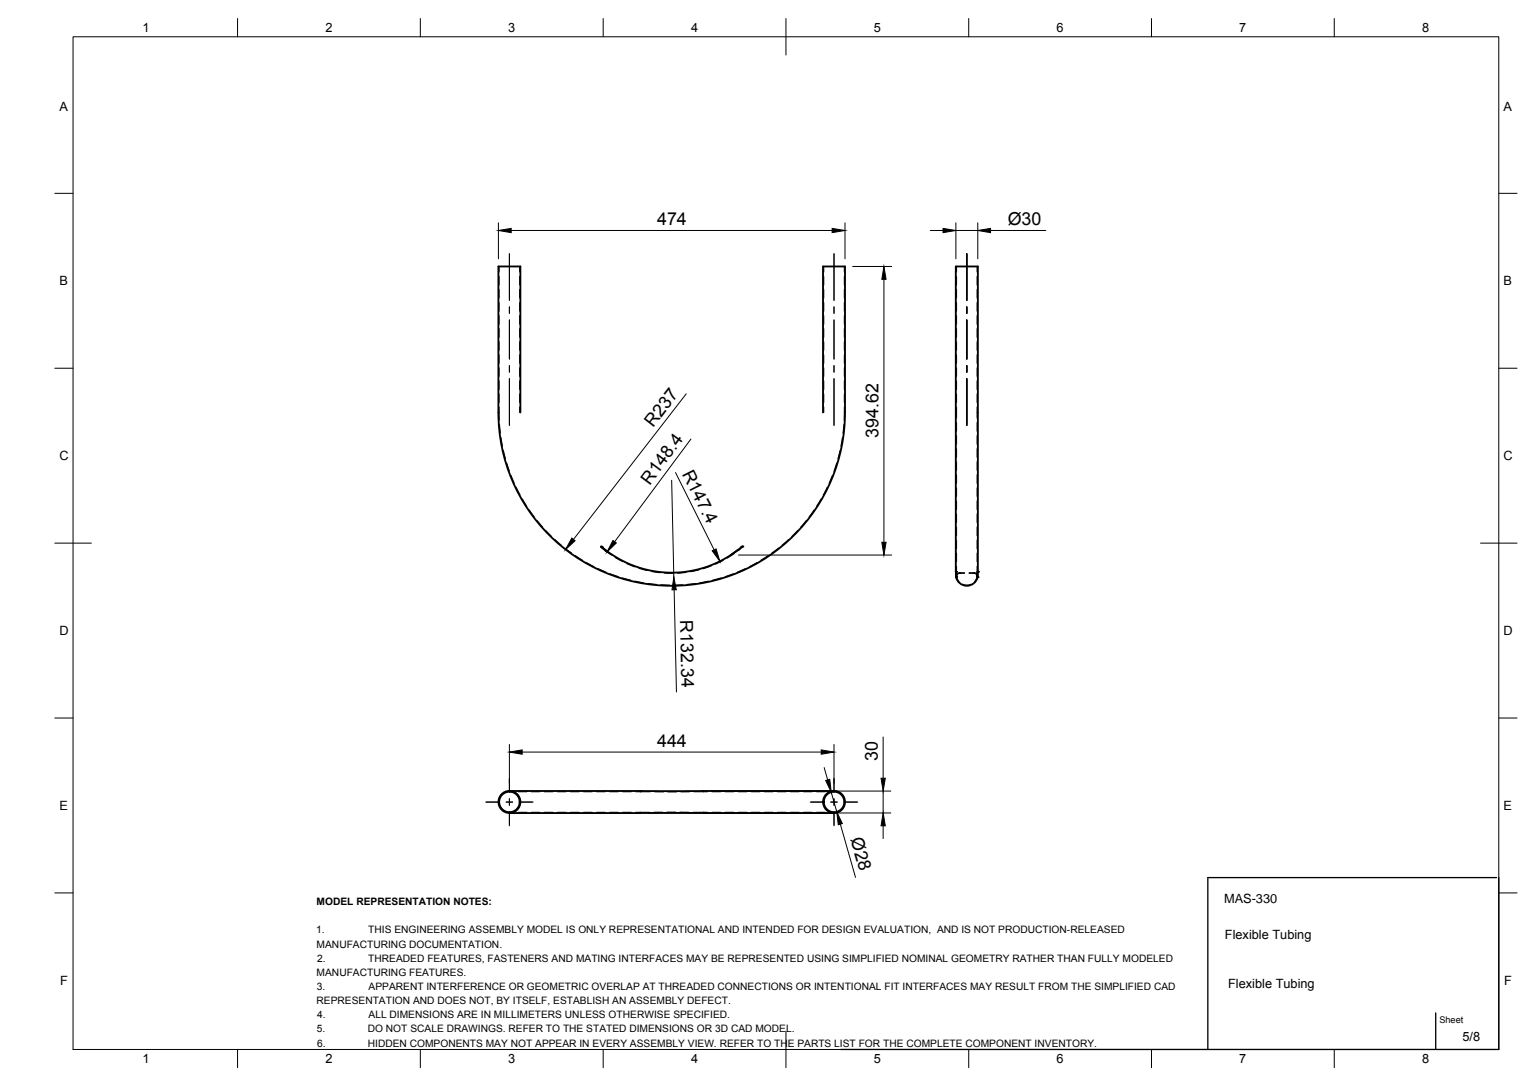
ISO-10303-21;
HEADER;
/* Generated by software containing ST-Developer
 * from STEP Tools, Inc. (www.steptools.com) 
 */

FILE_DESCRIPTION(
/* description */ ('STEP AP214'),
/* implementation_level */ '2;1');

FILE_NAME(
/* name */ 'Flexible Tubing.step',
/* time_stamp */ '2026-10-12T14:05:15-07:00',
/* author */ (''),
/* organization */ (''),
/* preprocessor_version */ 'ST-DEVELOPER v20.2',
/* originating_system */ 'Autodesk Translation Framework v15.15.0.0',
/* authorisation */ '');

FILE_SCHEMA (('AUTOMOTIVE_DESIGN { 1 0 10303 214 3 1 1 }'));
ENDSEC;

DATA;
#10=MECHANICAL_DESIGN_GEOMETRIC_PRESENTATION_REPRESENTATION('',(#284),#39959);
#184=(
BOUNDED_SURFACE()
B_SPLINE_SURFACE(3,2,((#27814,#27815,#27816),(#27817,#27818,#27819),(#27820,
#27821,#27822),(#27823,#27824,#27825),(#27826,#27827,#27828),(#27829,#27830,
#27831),(#27832,#27833,#27834),(#27835,#27836,#27837),(#27838,#27839,#27840),
(#27841,#27842,#27843),(#27844,#27845,#27846),(#27847,#27848,#27849),(#27850,
#27851,#27852),(#27853,#27854,#27855),(#27856,#27857,#27858),(#27859,#27860,
#27861),(#27862,#27863,#27864),(#27865,#27866,#27867),(#27868,#27869,#27870),
(#27871,#27872,#27873),(#27874,#27875,#27876),(#27877,#27878,#27879),(#27880,
#27881,#27882),(#27883,#27884,#27885),(#27886,#27887,#27888),(#27889,#27890,
#27891),(#27892,#27893,#27894),(#27895,#27896,#27897),(#27898,#27899,#27900),
(#27901,#27902,#27903),(#27904,#27905,#27906),(#27907,#27908,#27909),(#27910,
#27911,#27912),(#27913,#27914,#27915),(#27916,#27917,#27918),(#27919,#27920,
#27921),(#27922,#27923,#27924),(#27925,#27926,#27927),(#27928,#27929,#27930),
(#27931,#27932,#27933),(#27934,#27935,#27936),(#27937,#27938,#27939),(#27940,
#27941,#27942),(#27943,#27944,#27945),(#27946,#27947,#27948),(#27949,#27950,
#27951),(#27952,#27953,#27954),(#27955,#27956,#27957),(#27958,#27959,#27960),
(#27961,#27962,#27963),(#27964,#27965,#27966),(#27967,#27968,#27969),(#27970,
#27971,#27972),(#27973,#27974,#27975),(#27976,#27977,#27978),(#27979,#27980,
#27981),(#27982,#27983,#27984),(#27985,#27986,#27987),(#27988,#27989,#27990),
(#27991,#27992,#27993),(#27994,#27995,#27996),(#27997,#27998,#27999),(#28000,
#28001,#28002),(#28003,#28004,#28005),(#28006,#28007,#28008),(#28009,#28010,
#28011),(#28012,#28013,#28014),(#28015,#28016,#28017),(#28018,#28019,#28020),
(#28021,#28022,#28023),(#28024,#28025,#28026),(#28027,#28028,#28029),(#28030,
#28031,#28032),(#28033,#28034,#28035),(#28036,#28037,#28038),(#28039,#28040,
#28041),(#28042,#28043,#28044),(#28045,#28046,#28047),(#28048,#28049,#28050),
(#28051,#28052,#28053),(#28054,#28055,#28056),(#28057,#28058,#28059),(#28060,
#28061,#28062),(#28063,#28064,#28065),(#28066,#28067,#28068),(#28069,#28070,
#28071),(#28072,#28073,#28074),(#28075,#28076,#28077),(#28078,#28079,#28080),
(#28081,#28082,#28083),(#28084,#28085,#28086),(#28087,#28088,#28089),(#28090,
#28091,#28092),(#28093,#28094,#28095),(#28096,#28097,#28098),(#28099,#28100,
#28101)),.UNSPECIFIED.,.F.,.F.,.F.)
B_SPLINE_SURFACE_WITH_KNOTS((4,2,2,2,2,2,2,2,2,2,2,2,2,2,2,2,2,2,2,2,2,
2,2,2,2,2,2,2,2,2,2,2,2,2,2,2,2,2,2,2,2,2,2,2,2,2,2,4),(3,3),(0.22178007142157,
0.223701231496081,0.225435349569694,0.227169467643307,0.228036526680114,
0.228903585716921,0.229770644753727,0.230204174272131,0.230637703790534,
0.231071233308937,0.231504762827341,0.231938292345744,0.232371821864147,
0.232805351382551,0.233238880900954,0.234105939937761,0.234972998974567,
0.235840058011374,0.237574176084987,0.239308294158601,0.241042412232214,
0.242776530305827,0.246244766453054,0.249713002600281,0.256649474894734,
0.260117711041961,0.263585947189187,0.270522419483641,0.277458891778094,
0.291331836367001,0.298268308661454,0.305204780955908,0.319077725544815,
0.332950670133721,0.346823614722628,0.353760087017082,0.360696559311535,
0.374569503900442,0.388442448489349,0.402315393078255,0.409251865372709,
0.416188337667162,0.423124809961615,0.430061282256069,0.433529518403295,
0.436997754550522,0.440465990697749,0.444121268845909),(-0.000187042000933031,
1.00006570533259),.UNSPECIFIED.)
GEOMETRIC_REPRESENTATION_ITEM()
RATIONAL_B_SPLINE_SURFACE(((1.00001671480553,0.955315105954543,1.00000587097346),
(1.00001553678529,0.958464392346589,1.00000545720104),(1.00001436299837,
0.961602361500747,1.00000504491554),(1.00001214511377,0.96753159221984,
1.00000426589711),(1.0000110971902,0.970333081805704,1.00000389782035),
(1.00000903364032,0.975849718381431,1.00000317301105),(1.00000802454064,
0.978547417281528,1.00000281857094),(1.00000657099102,0.982433296228171,
1.0000023080205),(1.0000060954059,0.98370471220148,1.00000214097413),(1.0000051861456,
0.986135503257278,1.000001821602),(1.00000475111726,0.987298495868281,1.00000166880095),
(1.00000393900491,0.989469574341258,1.00000138355144),(1.00000355798186,
0.990488190713896,1.00000124971942),(1.00000307531353,0.991778542734027,
1.00000108018511),(1.00000292909575,0.992169437270804,1.00000102882701),
(1.00000267340501,0.992852993744571,1.0000009390172),(1.00000256420741,
0.993144919550281,1.00000090066221),(1.00000239821197,0.993588687122249,
1.00000084235732),(1.00000234012324,0.993743979916236,1.00000082195401),
(1.00000227962719,0.993905708377709,1.00000080070514),(1.00000227804363,
0.993909941827738,1.00000080014892),(1.00000233322191,0.993762429746366,
1.00000081952996),(1.00000238907502,0.993613113593466,1.00000083914802),
(1.00000255214859,0.993177157271913,1.00000089642662),(1.00000265990449,
0.992889085671756,1.00000093427522),(1.00000291128676,0.992217047317989,
1.00000102257171),(1.00000305564197,0.991831132138118,1.0000010732756),
(1.00000337449658,0.990978715127399,1.00000118527134),(1.00000355003229,
0.990509442879127,1.00000124692718),(1.00000410591494,0.98902336174389,
1.00000144217757),(1.00000451382822,0.987932857764997,1.00000158545462),
(1.0000053771532,0.985624868901155,1.00000188869225),(1.00000583381796,
0.984404034076013,1.00000204909296),(1.00000677789068,0.981880176447102,
1.00000238069275),(1.00000726052111,0.980589925744053,1.00000255021374),
(1.00000873064634,0.976659734042192,1.00000306658626),(1.00000973994235,
0.973961510289341,1.00000342109532),(1.00001179196766,0.968475683150999,
1.00000414185669),(1.00001283513645,0.96568690486921,1.00000450826337),
(1.00001494361968,0.960050144712234,1.00000524885524),(1.00001601138312,
0.95719561576597,1.00000562390063),(1.00001814845983,0.951482414616923,
1.00000637453578),(1.00001921796653,0.948623225275015,1.00000675019349),
(1.00002242616289,0.940046522775516,1.00000787705289),(1.00002456438731,
0.934330253373406,1.00000862809117),(1.00002882929853,0.922928558871327,
1.00001012611521),(1.00003095610456,0.91724281507434,1.00001087314285),
(1.00003730979308,0.900257041725582,1.00001310483718),(1.00004150973089,
0.889029045332982,1.00001458003971),(1.00004772883642,0.872403062390114,
1.00001676446258),(1.00004978850184,0.866896810424999,1.00001748790749),
(1.00005387724354,0.855966082598523,1.00001892405307),(1.00005590801946,
0.850537063013456,1.00001963735072),(1.00006192256307,0.834457950174723,
1.00002174992247),(1.00006583638793,0.823994840153908,1.00002312462957),
(1.00007345352895,0.803631388209101,1.00002580010388),(1.00007715685939,
0.793731008091671,1.0000271008761),(1.00008791765573,0.764963395833388,
1.00003088054016),(1.00009462794849,0.747024286693254,1.00003323748955),
(1.00010382896234,0.722426553366422,1.00003646928952),(1.00010675138937,
0.71461381858396,1.00003749577419),(1.00011227304363,0.699852382375851,
1.00003943522156),(1.00011487430917,0.692898231787275,1.00004034890021),
(1.00012212392104,0.673517321968125,1.00004289528215),(1.00012616942783,
0.662702177158641,1.00004431624172),(1.0001325032316,0.645769563161906,
1.00004654095165),(1.00013478994257,0.639656333948816,1.00004734414493),
(1.0001374601242,0.632517944987879,1.00004828202993),(1.00013784258632,
0.631495481447842,1.00004841636742),(1.00013694003487,0.63390833726827,
1.00004809935173),(1.00013639387768,0.635368418638627,1.00004790751735),
(1.00013481186227,0.63959773443293,1.00004735184409),(1.00013378125052,
0.642352943082953,1.000046989848),(1.00013001435257,0.652423262814007,1.00004566674808),
(1.00012660145365,0.661547211425516,1.00004446798815),(1.00011821711893,
0.683961657570758,1.00004152304174),(1.00011324709426,0.697248382663264,
1.0000397773509),(1.00010199064016,0.727341072498234,1.00003582359008),
(1.00009570502111,0.744144870834123,1.00003361580473),(1.00008544083,0.771584872526209,
1.00003001057023),(1.00008187300066,0.781123007795138,1.00002875739195),
(1.000074536318,0.800736690215974,1.00002618042693),(1.00007076318398,0.810823681264022,
1.00002485513662),(1.000063033788,0.831487232491117,1.00002214023345),(1.0000590774879,
0.84206389463353,1.00002075060717),(1.00005100479812,0.863645197935074,
1.00001791512414),(1.00004688833189,0.874650043707415,1.0000164692405),
(1.00004060950573,0.891435682115803,1.00001426384112),(1.00003849870446,
0.897078639254129,1.00001352243505),(1.00003426394995,0.908399713630422,
1.00001203500336),(1.00003213787031,0.914083515546979,1.00001128823086),
(1.00002787459407,0.925480839114136,1.00000979078109),(1.00002573731916,
0.931194570120134,1.00000904007632),(1.00002134529738,0.94293607843551,
1.00000749740547),(1.00001909036436,0.94896435336469,1.000006705374),(1.00001684310806,
0.954972105552579,1.00000591603894)))
REPRESENTATION_ITEM('')
SURFACE()
);
#185=(
BOUNDED_SURFACE()
B_SPLINE_SURFACE(3,2,((#28385,#28386,#28387),(#28388,#28389,#28390),(#28391,
#28392,#28393),(#28394,#28395,#28396),(#28397,#28398,#28399),(#28400,#28401,
#28402),(#28403,#28404,#28405),(#28406,#28407,#28408),(#28409,#28410,#28411),
(#28412,#28413,#28414),(#28415,#28416,#28417),(#28418,#28419,#28420),(#28421,
#28422,#28423),(#28424,#28425,#28426),(#28427,#28428,#28429),(#28430,#28431,
#28432),(#28433,#28434,#28435),(#28436,#28437,#28438),(#28439,#28440,#28441),
(#28442,#28443,#28444),(#28445,#28446,#28447),(#28448,#28449,#28450),(#28451,
#28452,#28453),(#28454,#28455,#28456),(#28457,#28458,#28459),(#28460,#28461,
#28462),(#28463,#28464,#28465),(#28466,#28467,#28468),(#28469,#28470,#28471),
(#28472,#28473,#28474),(#28475,#28476,#28477),(#28478,#28479,#28480),(#28481,
#28482,#28483),(#28484,#28485,#28486),(#28487,#28488,#28489),(#28490,#28491,
#28492),(#28493,#28494,#28495),(#28496,#28497,#28498),(#28499,#28500,#28501),
(#28502,#28503,#28504),(#28505,#28506,#28507),(#28508,#28509,#28510),(#28511,
#28512,#28513),(#28514,#28515,#28516),(#28517,#28518,#28519),(#28520,#28521,
#28522),(#28523,#28524,#28525),(#28526,#28527,#28528),(#28529,#28530,#28531),
(#28532,#28533,#28534),(#28535,#28536,#28537),(#28538,#28539,#28540),(#28541,
#28542,#28543),(#28544,#28545,#28546),(#28547,#28548,#28549),(#28550,#28551,
#28552),(#28553,#28554,#28555),(#28556,#28557,#28558),(#28559,#28560,#28561),
(#28562,#28563,#28564),(#28565,#28566,#28567),(#28568,#28569,#28570),(#28571,
#28572,#28573),(#28574,#28575,#28576),(#28577,#28578,#28579),(#28580,#28581,
#28582),(#28583,#28584,#28585),(#28586,#28587,#28588),(#28589,#28590,#28591),
(#28592,#28593,#28594),(#28595,#28596,#28597),(#28598,#28599,#28600),(#28601,
#28602,#28603),(#28604,#28605,#28606),(#28607,#28608,#28609),(#28610,#28611,
#28612),(#28613,#28614,#28615),(#28616,#28617,#28618),(#28619,#28620,#28621),
(#28622,#28623,#28624),(#28625,#28626,#28627),(#28628,#28629,#28630),(#28631,
#28632,#28633),(#28634,#28635,#28636),(#28637,#28638,#28639),(#28640,#28641,
#28642),(#28643,#28644,#28645),(#28646,#28647,#28648),(#28649,#28650,#28651),
(#28652,#28653,#28654),(#28655,#28656,#28657),(#28658,#28659,#28660),(#28661,
#28662,#28663),(#28664,#28665,#28666),(#28667,#28668,#28669),(#28670,#28671,
#28672),(#28673,#28674,#28675),(#28676,#28677,#28678),(#28679,#28680,#28681),
(#28682,#28683,#28684),(#28685,#28686,#28687),(#28688,#28689,#28690)),
 .UNSPECIFIED.,.F.,.F.,.F.)
B_SPLINE_SURFACE_WITH_KNOTS((4,2,2,2,2,2,2,2,2,2,2,2,2,2,2,2,2,2,2,2,2,
2,2,2,2,2,2,2,2,2,2,2,2,2,2,2,2,2,2,2,2,2,2,2,2,2,2,2,2,2,4),(3,3),(0.,
0.00173411807361341,0.00346823614722682,0.00520235422084023,0.00606941325764693,
0.00693647229445363,0.00780353133126034,0.00867059036806704,0.00910411988647039,
0.00953764940487375,0.0099711789232771,0.0104047084416805,0.0108382379600838,
0.0112717674784872,0.0117052969968905,0.0121388265152939,0.0130058855521006,
0.0138729445889073,0.0156070626625207,0.0173411807361341,0.0190752988097475,
0.0208094168833609,0.0242776530305877,0.0277458891778145,0.0346823614722682,
0.038150597619495,0.0416188337667218,0.0485553060611754,0.0554917783556291,
0.0693647229445363,0.0832376675334436,0.0867059036806704,0.0901741398278972,
0.0971106121223509,0.110983556711258,0.124856501300165,0.131792973594619,
0.135261209741846,0.138729445889073,0.15260239047798,0.166475335066887,
0.180348279655794,0.183816515803021,0.187284751950248,0.194221224244702,
0.201157696539155,0.208094168833609,0.211562404980836,0.215030641128063,
0.218498877275289,0.222038288720656),(0.,1.00007117529817),
 .UNSPECIFIED.)
GEOMETRIC_REPRESENTATION_ITEM()
RATIONAL_B_SPLINE_SURFACE(((1.,0.954058032824739,1.00000653986642),(1.,
0.956926189621845,1.00000613158259),(1.,0.959774945923169,1.00000572606044),
(1.,0.965414443781637,1.00000492327455),(1.,0.968205662454782,1.00000452594291),
(1.,0.973699562224279,1.000003743883),(1.,0.976403365991766,1.00000335899492),
(1.,0.98034605056057,1.00000279775142),(1.,0.981641163134558,1.00000261339138),
(1.,0.984176833060148,1.00000225243725),(1.,0.985416251002957,1.00000207600537),
(1.,0.987758111159059,1.00000174264018),(1.,0.988874643995945,1.00000158370106),
(1.,0.99087726268354,1.0000012986271),(1.,0.991757284799027,1.00000117335542),
(1.,0.992797059568252,1.00000102534287),(1.,0.993098523876015,1.00000098242924),
(1.,0.993562924435804,1.00000091632155),(1.,0.993726976585977,1.00000089296862),
(1.,0.9939034030842,1.00000086785421),(1.,0.993913510674876,1.00000086641539),
(1.,0.993776600284822,1.00000088590466),(1.,0.993631545571422,1.00000090655329),
(1.,0.993199734841636,1.0000009680218),(1.,0.992914845213595,1.00000100857601),
(1.,0.99224575536465,1.00000110382135),(1.,0.991859782611137,1.0000011587648),
(1.,0.991003776450707,1.00000128061779),(1.,0.990532224611597,1.00000134774347),
(1.,0.989541347388611,1.00000148879544),(1.,0.98901957113283,1.0000015630706),
(1.,0.987391710342441,1.00000179479755),(1.,0.986223928377901,1.00000196103201),
(1.,0.983775371631144,1.00000230958552),(1.,0.982504716794789,1.000002490464),
(1.,0.97863152044244,1.00000304181581),(1.,0.975951927850889,1.00000342325741),
(1.,0.970485088654407,1.00000420146523),(1.,0.967696119306073,1.00000459847668),
(1.,0.962047336054619,1.00000540258435),(1.,0.959183960598246,1.00000581018755),
(1.,0.953462458079452,1.00000662464684),(1.,0.950596652764379,1.00000703259594),
(1.,0.941994603975872,1.00000825710271),(1.,0.936254194204132,1.00000907425347),
(1.,0.924794890941365,1.00001070549212),(1.,0.919075593477731,1.00001151963753),
(1.,0.901978842716718,1.00001395337019),(1.,0.890663248710558,1.00001556415175),
(1.,0.8738935874927,1.00001795132302),(1.,0.868330212597956,1.00001874327276),
(1.,0.857329904873204,1.00002030917312),(1.,0.851890471291245,1.00002108347973),
(1.,0.835762777169572,1.00002337926661),(1.,0.825264842647475,1.00002487365385),
(1.,0.804827719776929,1.00002778289048),(1.,0.794888487743137,1.00002919774608),
(1.,0.765999443480927,1.00003331011876),(1.,0.747972792915185,1.00003587622322),
(1.,0.714994849965956,1.00004057065307),(1.,0.700044230979255,1.00004269888259),
(1.,0.683764200151961,1.00004501635469),(1.,0.680628844586273,1.00004546267443),
(1.,0.674640520726457,1.0000463151159),(1.,0.671783516007252,1.00004672181222),
(1.,0.663635510374337,1.00004788168568),(1.,0.658767677401333,1.00004857462461),
(1.,0.645945349063695,1.0000503998907),(1.,0.639777818633445,1.00005127784233),
(1.,0.632581312956382,1.00005230226921),(1.,0.631555065114158,1.0000524483562),
(1.,0.63399275055746,1.00005210135022),(1.,0.635466148812585,1.0000518916111),
(1.,0.638664401233599,1.00005143633796),(1.,0.639895676582775,1.00005126106518),
(1.,0.642669442581869,1.00005086621794),(1.,0.644213120868507,1.00005064647441),
(1.,0.652691129180967,1.00004943962487),(1.,0.661906311274784,1.00004812783821),
(1.,0.684528677277457,1.00004490753092),(1.,0.697932027791846,1.00004299955598),
(1.,0.728267963131221,1.00003868121749),(1.,0.745198393491031,1.00003627116063),
(1.,0.768222924620666,1.0000329936049),(1.,0.772921247385803,1.00003232479585),
(1.,0.782497618983893,1.00003096159364),(1.,0.787373779802698,1.00003026746924),
(1.,0.802194699878368,1.00002815770243),(1.,0.812351834256105,1.00002671182829),
(1.,0.833145675250053,1.00002375181263),(1.,0.843782502229831,1.00002223765397),
(1.,0.86547121370724,1.00001915025295),(1.,0.876523345831396,1.00001757697535),
(1.,0.893367253742941,1.00001517923502),(1.,0.899026187982997,1.00001437368235),
(1.,0.910424400977938,1.00001275113994),(1.,0.916164825311843,1.00001193398711),
(1.,0.927638312474702,1.00001030072937),(1.,0.933380131170828,1.00000948337806),
(1.,0.944959178856698,1.00000783509371),(1.,0.950796193416408,1.00000700419121),
(1.,0.95659226878001,1.00000617911642)))
REPRESENTATION_ITEM('')
SURFACE()
);
#186=(
BOUNDED_SURFACE()
B_SPLINE_SURFACE(3,2,((#29356,#29357,#29358),(#29359,#29360,#29361),(#29362,
#29363,#29364),(#29365,#29366,#29367),(#29368,#29369,#29370),(#29371,#29372,
#29373),(#29374,#29375,#29376),(#29377,#29378,#29379),(#29380,#29381,#29382),
(#29383,#29384,#29385),(#29386,#29387,#29388),(#29389,#29390,#29391),(#29392,
#29393,#29394),(#29395,#29396,#29397),(#29398,#29399,#29400),(#29401,#29402,
#29403),(#29404,#29405,#29406),(#29407,#29408,#29409),(#29410,#29411,#29412),
(#29413,#29414,#29415),(#29416,#29417,#29418),(#29419,#29420,#29421),(#29422,
#29423,#29424),(#29425,#29426,#29427),(#29428,#29429,#29430),(#29431,#29432,
#29433),(#29434,#29435,#29436),(#29437,#29438,#29439),(#29440,#29441,#29442),
(#29443,#29444,#29445),(#29446,#29447,#29448),(#29449,#29450,#29451),(#29452,
#29453,#29454),(#29455,#29456,#29457),(#29458,#29459,#29460),(#29461,#29462,
#29463),(#29464,#29465,#29466),(#29467,#29468,#29469),(#29470,#29471,#29472),
(#29473,#29474,#29475),(#29476,#29477,#29478),(#29479,#29480,#29481),(#29482,
#29483,#29484),(#29485,#29486,#29487),(#29488,#29489,#29490),(#29491,#29492,
#29493),(#29494,#29495,#29496),(#29497,#29498,#29499),(#29500,#29501,#29502),
(#29503,#29504,#29505),(#29506,#29507,#29508),(#29509,#29510,#29511),(#29512,
#29513,#29514),(#29515,#29516,#29517),(#29518,#29519,#29520),(#29521,#29522,
#29523),(#29524,#29525,#29526),(#29527,#29528,#29529),(#29530,#29531,#29532),
(#29533,#29534,#29535),(#29536,#29537,#29538),(#29539,#29540,#29541),(#29542,
#29543,#29544),(#29545,#29546,#29547),(#29548,#29549,#29550),(#29551,#29552,
#29553),(#29554,#29555,#29556),(#29557,#29558,#29559),(#29560,#29561,#29562),
(#29563,#29564,#29565),(#29566,#29567,#29568),(#29569,#29570,#29571),(#29572,
#29573,#29574),(#29575,#29576,#29577),(#29578,#29579,#29580),(#29581,#29582,
#29583),(#29584,#29585,#29586),(#29587,#29588,#29589),(#29590,#29591,#29592),
(#29593,#29594,#29595),(#29596,#29597,#29598),(#29599,#29600,#29601),(#29602,
#29603,#29604),(#29605,#29606,#29607),(#29608,#29609,#29610),(#29611,#29612,
#29613),(#29614,#29615,#29616),(#29617,#29618,#29619),(#29620,#29621,#29622),
(#29623,#29624,#29625),(#29626,#29627,#29628),(#29629,#29630,#29631),(#29632,
#29633,#29634),(#29635,#29636,#29637),(#29638,#29639,#29640),(#29641,#29642,
#29643)),.UNSPECIFIED.,.F.,.F.,.F.)
B_SPLINE_SURFACE_WITH_KNOTS((4,2,2,2,2,2,2,2,2,2,2,2,2,2,2,2,2,2,2,2,2,
2,2,2,2,2,2,2,2,2,2,2,2,2,2,2,2,2,2,2,2,2,2,2,2,2,2,4),(3,3),(0.221817496371262,
0.223701231496101,0.225435349569714,0.227169467643327,0.228036526680134,
0.228903585716941,0.229770644753747,0.23020417427215,0.230637703790554,
0.231071233308957,0.23150476282736,0.231938292345764,0.232371821864167,
0.23280535138257,0.233238880900974,0.23410593993778,0.234972998974587,0.235840058011393,
0.237574176085006,0.23930829415862,0.241042412232233,0.242776530305846,
0.246244766453072,0.249713002600299,0.256649474894752,0.260117711041978,
0.263585947189204,0.270522419483657,0.27745889177811,0.291331836367015,
0.298268308661468,0.305204780955921,0.319077725544826,0.332950670133732,
0.346823614722637,0.35376008701709,0.360696559311543,0.374569503900448,
0.388442448489354,0.402315393078259,0.409251865372712,0.416188337667165,
0.423124809961617,0.43006128225607,0.433529518403296,0.436997754550523,
0.440465990697749,0.44408384389623),(-0.000149617051253964,1.00007479383841),
 .UNSPECIFIED.)
GEOMETRIC_REPRESENTATION_ITEM()
RATIONAL_B_SPLINE_SURFACE(((1.00001331480133,0.955500401761319,1.00000665559565),
(1.00001239101105,0.958587815164465,1.00000619382575),(1.00001147053421,
0.961664154694889,1.00000573371211),(1.0000097146529,0.967532512098177,
1.00000485600949),(1.00000887643813,0.970333922314243,1.00000443701574),
(1.00000722584258,0.975850402594055,1.00000361194172),(1.00000641868232,
0.978548025065446,1.00000320847102),(1.00000525601474,0.982433793918799,
1.00000262729484),(1.00000487560295,0.983705173871199,1.00000243714052),
(1.00000414830239,0.986135896059087,1.00000207358883),(1.00000380033123,
0.98729885572081,1.00000189965042),(1.00000315073751,0.989469872683854,
1.00000157494163),(1.00000284596418,0.990488460197697,1.00000142259628),
(1.00000245988668,0.991778775660097,1.00000122960987),(1.00000234292976,
0.992169659122265,1.00000117114726),(1.00000213840745,0.992853196229914,
1.00000106891383),(1.0000020510623,0.993145113764892,1.0000010252531),(1.0000019182856,
0.993588868764268,1.00000095888275),(1.0000018718215,0.993744157158601,
1.000000935657),(1.00000182343182,0.993905881037986,1.00000091146872),(1.00000182216515,
0.993910114368128,1.00000091083556),(1.00000186630125,0.993762606465926,
1.00000093289762),(1.00000191097712,0.993613294543411,1.0000009552295),
(1.00000204141667,0.993177350573097,1.00000102043159),(1.00000212760863,
0.992889287134443,1.00000106351589),(1.00000232868468,0.992217267820518,
1.00000116402665),(1.00000244415175,0.991831363574199,1.00000122174454),
(1.00000269919769,0.990978970713684,1.00000134923293),(1.00000283960547,
0.990509711760598,1.00000141941779),(1.00000328424576,0.989023672728241,
1.00000164167766),(1.00000361052809,0.987933199644816,1.00000180477459),
(1.00000430108584,0.985625276169944,1.00000214995985),(1.00000466636358,
0.984404475932691,1.0000023325492),(1.00000542150997,0.981880689808502,
1.00000271002002),(1.00000580755716,0.980590475660211,1.00000290299128),
(1.00000698348326,0.976660395306211,1.00000349079492),(1.00000779080056,
0.973962247998255,1.00000389434413),(1.00000943217783,0.968476576281456,
1.00000471481025),(1.00001026658934,0.965687877010012,1.00000513190289),
(1.00001195312625,0.960051276550606,1.00000597494271),(1.00001280721057,
0.957196828477568,1.00000640186909),(1.00001451661888,0.951483789191777,
1.00000725634151),(1.00001537209761,0.948624680855099,1.0000076839649),
(1.00001793827481,0.940048221346092,1.00000896670562),(1.00001964860115,
0.934332113895509,1.00000982163693),(1.00002306002512,0.922930742418279,
1.00001152688645),(1.0000247612181,0.917245159708875,1.00001237725232),
(1.00002984341657,0.900259867589174,1.00001491766259),(1.0000332028695,
0.889032189306294,1.00001659693363),(1.00003817741751,0.872406677399274,
1.00001908353327),(1.00003982490596,0.866900581435969,1.00001990705415),
(1.00004309541517,0.855970163292049,1.00002154186539),(1.00004471979543,
0.850541297518764,1.00002235383532),(1.00004953071814,0.834462640227989,
1.00002475864448),(1.00005266131459,0.823999826640663,1.00002632351831),
(1.00005875412544,0.803636951622608,1.00002936909777),(1.00006171635128,
0.79373685199774,1.00003084980912),(1.00007032371416,0.764970054768136,
1.00003515232371),(1.00007569115378,0.747031453875889,1.00003783531589),
(1.00008305087536,0.722434417430132,1.00004151417897),(1.00008538847094,
0.714621904001906,1.00004268265986),(1.00008980514053,0.699860885997467,
1.00004489039591),(1.00009188584494,0.692906932438445,1.00004593046605),
(1.00009768467601,0.673526571699192,1.00004882909547),(1.0001009206024,
0.662711733315835,1.00005044661999),(1.00010598689542,0.645779599024357,
1.0000529790797),(1.00010781599343,0.639666543011674,1.00005389338074),
(1.00010995182255,0.632528356305523,1.00005496100576),(1.00011025774696,
0.631505921714365,1.00005511392649),(1.00010953581267,0.633918709193333,
1.00005475305721),(1.00010909895159,0.635378749188762,1.0000545346859),
(1.00010783352659,0.639607945165404,1.00005390214494),(1.00010700915923,
0.642363075750804,1.00005349007302),(1.00010399608691,0.652433110183563,
1.00005198394532),(1.00010126617189,0.661556800302084,1.00005061935789),
(1.00009455969692,0.683970611397211,1.00004726702956),(1.00009058426569,
0.697256960064698,1.00004527985287),(1.0000815804353,0.727348797329703,
1.00004077915827),(1.00007655268435,0.744152119587061,1.00003826596438),
(1.00006834254686,0.77159134386594,1.00003416200863),(1.00006548870585,
0.781129208903971,1.00003273547501),(1.00005962022847,0.800742335641159,
1.00002980203187),(1.00005660216804,0.810829040908275,1.0000282934108),
(1.0000504195665,0.831492006708402,1.00002520294817),(1.00004725499489,
0.842068369196021,1.00002362109137),(1.00004079779896,0.863649061069833,
1.00002039336876),(1.00003750511341,0.874653595057445,1.00001874747236),
(1.00003248279597,0.891438757903646,1.00001623699448),(1.00003079440489,
0.897081555169982,1.00001539302783),(1.00002740710273,0.908402308800912,
1.00001369983595),(1.00002570649076,0.914085949687904,1.0000128497605),
(1.00002229637459,0.925482950352643,1.00001114516471),(1.00002058680775,
0.931196519480498,1.00001029061304),(1.00001709216721,0.942876010290598,
1.00000854376652),(1.00001530696519,0.948842360878052,1.00000765140752),
(1.00001352770684,0.954788847051718,1.00000676201955)))
REPRESENTATION_ITEM('')
SURFACE()
);
#187=(
BOUNDED_SURFACE()
B_SPLINE_SURFACE(3,2,((#30000,#30001,#30002),(#30003,#30004,#30005),(#30006,
#30007,#30008),(#30009,#30010,#30011),(#30012,#30013,#30014),(#30015,#30016,
#30017),(#30018,#30019,#30020),(#30021,#30022,#30023),(#30024,#30025,#30026),
(#30027,#30028,#30029),(#30030,#30031,#30032),(#30033,#30034,#30035),(#30036,
#30037,#30038),(#30039,#30040,#30041),(#30042,#30043,#30044),(#30045,#30046,
#30047),(#30048,#30049,#30050),(#30051,#30052,#30053),(#30054,#30055,#30056),
(#30057,#30058,#30059),(#30060,#30061,#30062),(#30063,#30064,#30065),(#30066,
#30067,#30068),(#30069,#30070,#30071),(#30072,#30073,#30074),(#30075,#30076,
#30077),(#30078,#30079,#30080),(#30081,#30082,#30083),(#30084,#30085,#30086),
(#30087,#30088,#30089),(#30090,#30091,#30092),(#30093,#30094,#30095),(#30096,
#30097,#30098),(#30099,#30100,#30101),(#30102,#30103,#30104),(#30105,#30106,
#30107),(#30108,#30109,#30110),(#30111,#30112,#30113),(#30114,#30115,#30116),
(#30117,#30118,#30119),(#30120,#30121,#30122),(#30123,#30124,#30125),(#30126,
#30127,#30128),(#30129,#30130,#30131),(#30132,#30133,#30134),(#30135,#30136,
#30137),(#30138,#30139,#30140),(#30141,#30142,#30143),(#30144,#30145,#30146),
(#30147,#30148,#30149),(#30150,#30151,#30152),(#30153,#30154,#30155),(#30156,
#30157,#30158),(#30159,#30160,#30161),(#30162,#30163,#30164),(#30165,#30166,
#30167),(#30168,#30169,#30170),(#30171,#30172,#30173),(#30174,#30175,#30176),
(#30177,#30178,#30179),(#30180,#30181,#30182),(#30183,#30184,#30185),(#30186,
#30187,#30188),(#30189,#30190,#30191),(#30192,#30193,#30194),(#30195,#30196,
#30197),(#30198,#30199,#30200),(#30201,#30202,#30203),(#30204,#30205,#30206),
(#30207,#30208,#30209),(#30210,#30211,#30212),(#30213,#30214,#30215),(#30216,
#30217,#30218),(#30219,#30220,#30221),(#30222,#30223,#30224),(#30225,#30226,
#30227),(#30228,#30229,#30230),(#30231,#30232,#30233),(#30234,#30235,#30236),
(#30237,#30238,#30239),(#30240,#30241,#30242),(#30243,#30244,#30245),(#30246,
#30247,#30248),(#30249,#30250,#30251),(#30252,#30253,#30254),(#30255,#30256,
#30257),(#30258,#30259,#30260),(#30261,#30262,#30263),(#30264,#30265,#30266),
(#30267,#30268,#30269),(#30270,#30271,#30272),(#30273,#30274,#30275),(#30276,
#30277,#30278),(#30279,#30280,#30281),(#30282,#30283,#30284),(#30285,#30286,
#30287),(#30288,#30289,#30290),(#30291,#30292,#30293),(#30294,#30295,#30296),
(#30297,#30298,#30299)),.UNSPECIFIED.,.F.,.F.,.F.)
B_SPLINE_SURFACE_WITH_KNOTS((4,2,2,2,2,2,2,2,2,2,2,2,2,2,2,2,2,2,2,2,2,
2,2,2,2,2,2,2,2,2,2,2,2,2,2,2,2,2,2,2,2,2,2,2,2,2,2,2,2,4),(3,3),(-0.000102234541641357,
0.00346823614722661,0.00520235422083992,0.00606941325764658,0.00693647229445323,
0.00780353133125988,0.00867059036806653,0.00910411988646986,0.00953764940487319,
0.00997117892327651,0.0104047084416798,0.0108382379600832,0.0112717674784865,
0.0117052969968898,0.0121388265152932,0.0130058855520998,0.0138729445889065,
0.0156070626625198,0.0173411807361331,0.0190752988097464,0.0208094168833597,
0.0242776530305863,0.0277458891778129,0.0346823614722661,0.0381505976194928,
0.0416188337667194,0.0485553060611726,0.0554917783556258,0.0693647229445323,
0.0832376675334387,0.0867059036806654,0.090174139827892,0.0971106121223452,
0.110983556711252,0.124856501300158,0.131792973594611,0.135261209741838,
0.138729445889065,0.152602390477971,0.166475335066877,0.180348279655784,
0.183816515803011,0.187284751950237,0.19422122424469,0.201157696539144,
0.208094168833597,0.211562404980823,0.21503064112805,0.218498877275277,
0.22202653747512),(0.,1.00010223454164),.UNSPECIFIED.)
GEOMETRIC_REPRESENTATION_ITEM()
RATIONAL_B_SPLINE_SURFACE(((1.,0.953549407570009,1.00000949771005),(1.,
0.959455865791245,1.00000829002195),(1.,0.965295688977991,1.00000709595866),
(1.,0.973698745410201,1.00000537779342),(1.,0.976402633150356,1.00000482493197),
(1.,0.980345440167197,1.00000401874983),(1.,0.981640592963782,1.00000375393113),
(1.,0.9841763416393,1.00000323544892),(1.,0.985415798074981,1.0000029820184),
(1.,0.987757730962312,1.00000250316553),(1.,0.988874298475363,1.00000227486199),
(1.,0.990876979358417,1.00000186537567),(1.,0.991757028804683,1.00000168543276),
(1.,0.992796835866325,1.00000147282437),(1.,0.993098309536668,1.00000141118232),
(1.,0.99356272451931,1.00000131622382),(1.,0.993726781764482,1.00000128267918),
(1.,0.993903213741988,1.0000012466043),(1.,0.993913321646593,1.00000124453754),
(1.,0.993776407004476,1.00000127253235),(1.,0.993631347786124,1.00000130219248),
(1.,0.993199523645578,1.00000139048717),(1.,0.992914625169687,1.0000014487401),
(1.,0.992245514540845,1.00000158555253),(1.,0.99185952980013,1.00000166447448),
(1.,0.991003497054706,1.00000183950671),(1.,0.990531930570611,1.00000193592748),
(1.,0.989541022573869,1.00000213853753),(1.,0.989019230113308,1.00000224522795),
(1.,0.987391318766343,1.00000257808549),(1.,0.986223500534092,1.00000281686822),
(1.,0.983774867742231,1.00000331753792),(1.,0.982504173443108,1.00000357735562),
(1.,0.978630856801064,1.00000436932912),(1.,0.975951180989188,1.00000491723998),
(1.,0.970484172008772,1.00000603507429),(1.,0.96769511604352,1.00000660535001),
(1.,0.96204615735736,1.00000776038741),(1.,0.959182692973428,1.00000834587735),
(1.,0.953461012761225,1.00000951578406),(1.,0.950595118442744,1.00001010177084),
(1.,0.941992802500896,1.0000118606785),(1.,0.936252214448483,1.00001303445127),
(1.,0.924792555293885,1.00001537759728),(1.,0.919073080205329,1.0000165470531),
(1.,0.901975798471311,1.00002004291863),(1.,0.890659853037534,1.00002235667962),
(1.,0.873889671000668,1.00002578566336),(1.,0.868326123324781,1.00002692323686),
(1.,0.857325473963624,1.00002917252955),(1.,0.851885871450147,1.00003028476009),
(1.,0.83575767644592,1.00003358247733),(1.,0.825259415892199,1.00003572904704),
(1.,0.804821658304747,1.0000399079366),(1.,0.794882117587898,1.00004194026538),
(1.,0.765992176118451,1.00004784736523),(1.,0.74796496570046,1.00005153337242),
(1.,0.714985998549083,1.0000582765516),(1.,0.700034915249734,1.0000613335859),
(1.,0.683754378804637,1.00006466245226),(1.,0.680618925863469,1.00006530355545),
(1.,0.674630416028701,1.00006652802056),(1.,0.671773322578567,1.00006711220784),
(1.,0.663625063888358,1.00006877827483),(1.,0.658757079736063,1.00006977362708),
(1.,0.645934353180302,1.00007239547823),(1.,0.63976663119061,1.00007365658669),
(1.,0.632569902032773,1.0000751280953),(1.,0.631543622312258,1.00007533793778),
(1.,0.633981383455941,1.00007483949099),(1.,0.63545482746786,1.00007453821724),
(1.,0.638653179224426,1.00007388425319),(1.,0.639884492811753,1.00007363248763),
(1.,0.642658344954122,1.00007306532063),(1.,0.644202071179115,1.00007274967634),
(1.,0.652680342816058,1.00007101613191),(1.,0.661895811073965,1.00006913185356),
(1.,0.684518879688121,1.00006450613546),(1.,0.697922646449475,1.00006176547956),
(1.,0.728259523947718,1.00005556252603),(1.,0.745190480114726,1.00005210066894),
(1.,0.768215726310939,1.00004739271796),(1.,0.772914194992678,1.00004643202638),
(1.,0.782490864005998,1.00004447389364),(1.,0.787367176263245,1.00004347683855),
(1.,0.802188556632332,1.00004044632449),(1.,0.81234600646155,1.00003836944003),
(1.,0.833140493248966,1.00003411761038),(1.,0.843777650575237,1.00003194264058),
(1.,0.865467035644792,1.00002750783189),(1.,0.876519511015255,1.00002524794239),
(1.,0.893363942044945,1.00002180377701),(1.,0.899023052036312,1.00002064666398),
(1.,0.910421619025157,1.00001831600944),(1.,0.916162221641087,1.00001714223369),
(1.,0.927636065134229,1.00001479618742),(1.,0.933378062154726,1.00001362212656),
(1.,0.944938051744135,1.00001125846608),(1.,0.950755904868764,1.00001006889499),
(1.,0.956533186645504,1.00000888761948)))
REPRESENTATION_ITEM('')
SURFACE()
);
#270=SHAPE_REPRESENTATION_RELATIONSHIP('SRR','None',#40004,#277);
#277=ADVANCED_BREP_SHAPE_REPRESENTATION('',(#292),#39954);
#284=STYLED_ITEM('',(#40046),#292);
#292=MANIFOLD_SOLID_BREP('Body1',#18261);
#389=PLANE('',#18748);
#390=PLANE('',#18749);
#954=FACE_BOUND('',#6088,.T.);
#955=FACE_BOUND('',#6090,.T.);
#1106=B_SPLINE_CURVE_WITH_KNOTS('',3,(#27167,#27168,#27169,#27170,#27171,
#27172,#27173,#27174,#27175,#27176,#27177,#27178,#27179,#27180,#27181,#27182,
#27183,#27184,#27185,#27186,#27187,#27188,#27189,#27190,#27191,#27192,#27193,
#27194,#27195,#27196,#27197,#27198,#27199,#27200,#27201,#27202,#27203,#27204,
#27205,#27206,#27207,#27208,#27209,#27210,#27211,#27212,#27213,#27214,#27215,
#27216,#27217,#27218,#27219,#27220,#27221,#27222,#27223,#27224,#27225,#27226,
#27227,#27228,#27229,#27230,#27231,#27232,#27233,#27234,#27235,#27236,#27237,
#27238,#27239,#27240,#27241,#27242,#27243,#27244,#27245,#27246,#27247,#27248,
#27249,#27250,#27251,#27252,#27253,#27254,#27255,#27256,#27257,#27258,#27259,
#27260,#27261,#27262,#27263,#27264,#27265,#27266),.UNSPECIFIED.,.F.,.F.,
(4,3,3,3,3,3,3,3,3,3,3,3,3,3,3,3,3,3,3,3,3,3,3,3,3,3,3,3,3,3,3,3,3,4),(0.460209507152456,
0.461151420671335,0.462093334190213,0.462902601160825,0.462955010568935,
0.463641386423054,0.464002099657692,0.464327762277174,0.464886176252622,
0.465429272087291,0.465700513985413,0.465946575674178,0.466383479195188,
0.466806080207127,0.466953830111869,0.467073265693652,0.467448107915379,
0.467815545281024,0.467998655841874,0.468322253700499,0.468446017401892,
0.468744114624328,0.469031905032931,0.469096950144427,0.469132393256011,
0.469479983587368,0.469671620413561,0.469818769110131,0.470094277283303,
0.470264386451509,0.470633430176549,0.4708701753027,0.471160215519294,0.47119152081837),
 .UNSPECIFIED.);
#1107=B_SPLINE_CURVE_WITH_KNOTS('',3,(#27268,#27269,#27270,#27271,#27272,
#27273,#27274,#27275,#27276,#27277,#27278,#27279,#27280,#27281,#27282,#27283,
#27284,#27285,#27286,#27287,#27288,#27289,#27290,#27291,#27292,#27293,#27294,
#27295,#27296,#27297,#27298,#27299,#27300,#27301,#27302,#27303,#27304,#27305,
#27306,#27307,#27308,#27309,#27310,#27311,#27312,#27313,#27314,#27315,#27316,
#27317,#27318,#27319,#27320,#27321,#27322,#27323,#27324,#27325,#27326,#27327,
#27328,#27329,#27330,#27331,#27332,#27333,#27334,#27335,#27336,#27337,#27338,
#27339,#27340,#27341,#27342,#27343,#27344,#27345),.UNSPECIFIED.,.F.,.F.,
(4,2,2,2,2,2,2,2,2,2,2,2,2,2,2,2,2,2,2,2,2,2,2,2,2,2,2,2,2,2,2,2,2,2,2,
2,2,2,4),(0.238679919152522,0.239545269105647,0.240410619058772,0.241275969011897,
0.242141318965021,0.243872018871271,0.24560271877752,0.24733341868377,0.249064118590019,
0.252525518402518,0.255986918215017,0.259448318027516,0.266371117652514,
0.269832517465013,0.273293917277512,0.28021671690251,0.294062316152505,
0.307907915402501,0.314830715027499,0.318292114839998,0.321753514652497,
0.335599113902493,0.349444713152489,0.363290312402485,0.366751712214984,
0.370213112027483,0.377135911652481,0.390981510902477,0.404827110152473,
0.418672709402469,0.422134109214968,0.425595509027467,0.432518308652464,
0.439441108277462,0.44636390790246,0.449825307714959,0.453286707527458,
0.456748107339957,0.460209507152456),.UNSPECIFIED.);
#1108=B_SPLINE_CURVE_WITH_KNOTS('',3,(#27352,#27353,#27354,#27355,#27356,
#27357,#27358,#27359,#27360,#27361,#27362,#27363,#27364,#27365,#27366,#27367),
 .UNSPECIFIED.,.F.,.F.,(4,2,2,2,2,2,2,4),(0.227148662184115,0.230031476426217,
0.232914290668319,0.23435569778937,0.235797104910421,0.237238512031472,
0.237959215591997,0.238679919152522),.UNSPECIFIED.);
#1109=B_SPLINE_CURVE_WITH_KNOTS('',3,(#27368,#27369,#27370,#27371,#27372,
#27373,#27374,#27375,#27376,#27377,#27378,#27379,#27380,#27381,#27382,#27383,
#27384,#27385,#27386,#27387,#27388,#27389,#27390,#27391,#27392,#27393,#27394,
#27395,#27396,#27397,#27398,#27399,#27400,#27401,#27402,#27403,#27404,#27405,
#27406,#27407,#27408,#27409,#27410,#27411,#27412,#27413,#27414,#27415,#27416,
#27417,#27418,#27419,#27420,#27421,#27422,#27423,#27424,#27425,#27426,#27427,
#27428,#27429,#27430,#27431,#27432,#27433,#27434,#27435,#27436,#27437,#27438,
#27439,#27440,#27441,#27442,#27443,#27444,#27445),.UNSPECIFIED.,.F.,.F.,
(4,2,2,2,2,2,2,2,2,2,2,2,2,2,2,2,2,2,2,2,2,2,2,2,2,2,2,2,2,2,2,2,2,2,2,
2,2,2,4),(0.00739566262098398,0.00825407277552746,0.00911248293007093,0.00997089308461441,
0.0108293032391579,0.0116877133937014,0.0125461235482448,0.0142629438573318,
0.0176965844755058,0.0194134047845928,0.0211302250936798,0.0245638657118537,
0.0279975063300277,0.0348647875663756,0.0382984281845495,0.0417320688027234,
0.0485993500390712,0.0623339125117668,0.0760684749844625,0.0829357562208103,
0.0863693968389842,0.0898030374571581,0.103537599929854,0.117272162402549,
0.131006724875245,0.137874006111593,0.144741287347941,0.158475849820636,
0.172210412293332,0.185944974766028,0.189378615384202,0.192812256002376,
0.199679537238724,0.206546818475071,0.213414099711419,0.216847740329593,
0.220281380947767,0.223715021565941,0.227148662184115),.UNSPECIFIED.);
#1110=B_SPLINE_CURVE_WITH_KNOTS('',3,(#27455,#27456,#27457,#27458,#27459,
#27460,#27461,#27462,#27463,#27464,#27465,#27466,#27467,#27468,#27469,#27470,
#27471,#27472,#27473,#27474,#27475,#27476,#27477,#27478,#27479,#27480,#27481,
#27482,#27483,#27484,#27485,#27486,#27487,#27488,#27489,#27490,#27491,#27492,
#27493,#27494,#27495,#27496,#27497,#27498,#27499,#27500,#27501,#27502,#27503,
#27504,#27505,#27506,#27507,#27508,#27509,#27510,#27511,#27512,#27513,#27514,
#27515,#27516,#27517,#27518,#27519,#27520,#27521,#27522,#27523,#27524,#27525,
#27526,#27527,#27528,#27529,#27530),.UNSPECIFIED.,.F.,.F.,(4,2,2,2,2,2,
2,2,2,2,2,2,2,2,2,2,2,2,2,2,2,2,2,2,2,2,2,2,2,2,2,2,2,2,2,2,2,4),(0.00794038585254472,
0.00880514189733557,0.00966989794212641,0.0105346539869173,0.0113994100317081,
0.0122641660764989,0.0131289221212898,0.0148584342108715,0.0183174583900349,
0.0217764825691984,0.0252355067483618,0.0286945309275253,0.0356125792858521,
0.0390716034650155,0.0425306276441789,0.0494486760025058,0.0632847727191596,
0.0771208694358133,0.0840389177941402,0.0909569661524671,0.104793062869121,
0.118629159585775,0.132465256302429,0.135924280481592,0.139383304660755,
0.146301353019082,0.160137449735736,0.17397354645239,0.187809643169044,
0.191268667348207,0.19472769152737,0.201645739885697,0.208563788244024,
0.215481836602351,0.218940860781514,0.222399884960678,0.225858909139841,
0.229317933319005),.UNSPECIFIED.);
#1111=B_SPLINE_CURVE_WITH_KNOTS('',3,(#27532,#27533,#27534,#27535,#27536,
#27537,#27538,#27539,#27540,#27541,#27542,#27543,#27544,#27545,#27546,#27547,
#27548,#27549,#27550,#27551,#27552,#27553,#27554,#27555,#27556,#27557,#27558,
#27559,#27560,#27561,#27562,#27563,#27564,#27565,#27566,#27567,#27568,#27569,
#27570,#27571,#27572,#27573,#27574,#27575,#27576,#27577,#27578,#27579,#27580,
#27581,#27582,#27583,#27584,#27585,#27586,#27587,#27588,#27589,#27590,#27591,
#27592,#27593,#27594,#27595,#27596,#27597,#27598,#27599,#27600,#27601,#27602,
#27603,#27604,#27605,#27606,#27607,#27608,#27609,#27610,#27611,#27612,#27613,
#27614,#27615,#27616,#27617,#27618,#27619,#27620,#27621,#27622,#27623,#27624,
#27625,#27626,#27627,#27628),.UNSPECIFIED.,.F.,.F.,(4,3,3,3,3,3,3,3,3,3,
3,3,3,3,3,3,3,3,3,3,3,3,3,3,3,3,3,3,3,3,3,3,4),(0.229317933319005,0.230219578872938,
0.231090137167458,0.2312226752802,0.231993548591037,0.232168511536746,0.232709951257979,
0.233162059154581,0.233593800645616,0.234128304964287,0.23464985746595,
0.235019089754487,0.235170367762224,0.235605699057557,0.236029101015188,
0.236218790613006,0.236444378863357,0.236828028579282,0.237209220341014,
0.237314371101707,0.237650300518339,0.237869667972228,0.238217872028818,
0.238476872425152,0.238822259812058,0.239089125159825,0.239294957081098,
0.239577620782566,0.239723674920968,0.240110911517401,0.240374392336933,
0.240670477938072,0.240720246189969),.UNSPECIFIED.);
#1112=B_SPLINE_CURVE_WITH_KNOTS('',3,(#27635,#27636,#27637,#27638,#27639,
#27640,#27641,#27642,#27643,#27644,#27645,#27646,#27647,#27648,#27649,#27650,
#27651,#27652,#27653,#27654,#27655,#27656,#27657,#27658,#27659,#27660,#27661,
#27662,#27663,#27664,#27665,#27666,#27667,#27668,#27669,#27670,#27671,#27672,
#27673,#27674,#27675,#27676,#27677,#27678,#27679,#27680,#27681,#27682,#27683,
#27684,#27685,#27686,#27687,#27688,#27689,#27690,#27691,#27692,#27693,#27694,
#27695,#27696,#27697,#27698,#27699,#27700,#27701,#27702,#27703,#27704,#27705,
#27706,#27707,#27708,#27709,#27710),.UNSPECIFIED.,.F.,.F.,(4,2,2,2,2,2,
2,2,2,2,2,2,2,2,2,2,2,2,2,2,2,2,2,2,2,2,2,2,2,2,2,2,2,2,2,2,2,4),(0.240720246189969,
0.241587257099786,0.242454268009604,0.244188289829239,0.245055300739056,
0.245922311648874,0.247656333468509,0.251124377107779,0.252858398927414,
0.254592420747049,0.258060464386319,0.261528508025589,0.268464595304129,
0.271932638943399,0.275400682582669,0.282336769861209,0.29620894441829,
0.31008111897537,0.31701720625391,0.32048524989318,0.32395329353245,0.33782546808953,
0.351697642646611,0.365569817203691,0.372505904482231,0.379441991760771,
0.393314166317851,0.407186340874931,0.421058515432011,0.424526559071281,
0.427994602710552,0.434930689989092,0.441866777267632,0.448802864546172,
0.452270908185442,0.455738951824712,0.459206995463982,0.462675039103252),
 .UNSPECIFIED.);
#1113=B_SPLINE_CURVE_WITH_KNOTS('',3,(#27711,#27712,#27713,#27714,#27715,
#27716,#27717,#27718,#27719,#27720,#27721,#27722,#27723,#27724,#27725,#27726,
#27727,#27728,#27729,#27730,#27731,#27732,#27733,#27734,#27735,#27736,#27737,
#27738,#27739,#27740,#27741,#27742,#27743,#27744,#27745,#27746,#27747,#27748,
#27749,#27750,#27751,#27752,#27753,#27754,#27755,#27756,#27757,#27758,#27759,
#27760,#27761,#27762,#27763,#27764,#27765,#27766,#27767,#27768,#27769,#27770,
#27771,#27772,#27773,#27774,#27775,#27776,#27777,#27778,#27779,#27780,#27781,
#27782,#27783,#27784,#27785,#27786,#27787,#27788,#27789,#27790,#27791,#27792,
#27793,#27794,#27795,#27796,#27797,#27798,#27799,#27800,#27801,#27802,#27803,
#27804,#27805,#27806,#27807,#27808,#27809,#27810,#27811,#27812,#27813),
 .UNSPECIFIED.,.F.,.F.,(4,3,3,3,3,3,3,3,3,3,3,3,3,3,3,3,3,3,3,3,3,3,3,3,
3,3,3,3,3,3,3,3,3,3,4),(0.462675039103252,0.463642750480073,0.46457571174879,
0.465419810646746,0.465637485084959,0.466378096580386,0.46650737588057,
0.466828801914374,0.467118708075813,0.467646311136065,0.46816291669427,
0.468463738208056,0.468599931066666,0.469042894113483,0.4694858571603,0.469885588555766,
0.47008115405752,0.470495888471532,0.470551832133678,0.470927952128342,
0.471304862088803,0.471562377048373,0.471673225717309,0.471998870547497,
0.472322619053715,0.472644470724174,0.472868538651809,0.473043600039227,
0.473311697268788,0.473502563110719,0.473784211534654,0.474111751611527,
0.474153415877385,0.474442628569102,0.474524823030081),.UNSPECIFIED.);
#1114=B_SPLINE_CURVE_WITH_KNOTS('',3,(#28104,#28105,#28106,#28107,#28108,
#28109,#28110,#28111,#28112,#28113,#28114,#28115,#28116,#28117,#28118,#28119,
#28120,#28121,#28122,#28123,#28124,#28125,#28126,#28127,#28128,#28129,#28130,
#28131,#28132,#28133,#28134,#28135,#28136,#28137,#28138,#28139,#28140,#28141,
#28142,#28143,#28144,#28145,#28146,#28147,#28148,#28149,#28150,#28151,#28152,
#28153,#28154,#28155,#28156,#28157,#28158,#28159,#28160,#28161,#28162,#28163,
#28164,#28165,#28166,#28167,#28168,#28169,#28170,#28171,#28172,#28173,#28174,
#28175,#28176,#28177,#28178,#28179,#28180,#28181,#28182,#28183,#28184,#28185,
#28186,#28187,#28188,#28189,#28190,#28191,#28192,#28193,#28194,#28195,#28196,
#28197,#28198,#28199,#28200,#28201,#28202,#28203,#28204,#28205,#28206,#28207,
#28208,#28209,#28210,#28211,#28212,#28213,#28214,#28215,#28216,#28217,#28218,
#28219,#28220,#28221,#28222,#28223,#28224,#28225,#28226,#28227,#28228,#28229,
#28230,#28231,#28232,#28233,#28234,#28235,#28236,#28237,#28238,#28239,#28240,
#28241,#28242,#28243,#28244,#28245,#28246,#28247,#28248,#28249,#28250,#28251,
#28252,#28253,#28254,#28255,#28256,#28257,#28258,#28259,#28260,#28261,#28262,
#28263,#28264,#28265,#28266,#28267,#28268,#28269,#28270,#28271,#28272,#28273,
#28274,#28275,#28276,#28277,#28278,#28279,#28280,#28281,#28282,#28283,#28284,
#28285,#28286,#28287,#28288,#28289,#28290,#28291,#28292,#28293,#28294,#28295,
#28296,#28297,#28298,#28299,#28300,#28301,#28302,#28303,#28304,#28305,#28306,
#28307,#28308,#28309,#28310,#28311,#28312,#28313,#28314,#28315,#28316,#28317,
#28318,#28319,#28320,#28321,#28322,#28323,#28324,#28325,#28326,#28327,#28328,
#28329,#28330,#28331,#28332,#28333,#28334,#28335,#28336,#28337,#28338,#28339,
#28340,#28341,#28342,#28343,#28344,#28345,#28346,#28347,#28348,#28349,#28350,
#28351,#28352,#28353,#28354,#28355,#28356,#28357,#28358,#28359,#28360,#28361,
#28362,#28363,#28364,#28365,#28366,#28367,#28368,#28369,#28370,#28371,#28372,
#28373,#28374),.UNSPECIFIED.,.F.,.F.,(4,3,3,3,3,3,3,3,3,3,3,3,3,3,3,3,3,
3,3,3,3,3,3,3,3,3,3,3,3,3,3,3,3,3,3,3,3,3,3,3,3,3,3,3,3,3,3,3,3,3,3,3,3,
3,3,3,3,3,3,3,3,3,3,3,3,3,3,3,3,3,3,3,3,3,3,3,3,3,3,3,3,3,3,3,3,3,3,3,3,
3,4),(0.224444858500095,0.22692744060886,0.227879496390915,0.230926240713455,
0.231314134281736,0.235244024646494,0.238183410063376,0.244065722262328,
0.245052685845016,0.250738517111399,0.251921961626656,0.256859015714205,
0.258791237408296,0.261072409990444,0.26336646159019,0.265660513189936,
0.269986768381055,0.2743274185893,0.278683851522941,0.279399064753217,0.283831667173853,
0.288484641745175,0.293137616316497,0.297522480509796,0.301898066219627,
0.306256408549942,0.306876167879778,0.312710660889063,0.313745443661418,
0.318006273157165,0.320614719443058,0.324985848032814,0.329367820397019,
0.333760180874338,0.334353271006338,0.338776399740954,0.343198036678773,
0.347612751200278,0.348091822569619,0.352412228570066,0.356719848561029,
0.361005562897052,0.361830374132899,0.365456509513952,0.36869964991454,
0.37311710254083,0.37556892569618,0.380066366428911,0.384686921844185,0.38930747725946,
0.393839857281756,0.398442943052248,0.403046028822741,0.404952521931736,
0.406480666713561,0.409915304604381,0.413625500232383,0.416784580386021,
0.419769424576158,0.420219218276841,0.422728197517123,0.423653856167661,
0.425371175113071,0.426528854434269,0.427088494058482,0.428483134892337,
0.428805813003892,0.429979788180236,0.430523131949302,0.431264106069434,
0.432038976771861,0.432240450894712,0.433018232487655,0.433099110367417,
0.433957769840122,0.434387099576474,0.434816429312827,0.435245759049179,
0.435675088785532,0.436104418521884,0.436533748258237,0.437164180274058,
0.437392407730942,0.438251067203647,0.43897915760757,0.439109726676352,
0.440209087477563,0.440827045621762,0.441983333957617,0.442544364567172,
0.444261683512582),.UNSPECIFIED.);
#1115=B_SPLINE_CURVE_WITH_KNOTS('',3,(#28693,#28694,#28695,#28696,#28697,
#28698,#28699,#28700,#28701,#28702,#28703,#28704,#28705,#28706,#28707,#28708,
#28709,#28710,#28711,#28712,#28713,#28714,#28715,#28716,#28717,#28718,#28719,
#28720,#28721,#28722,#28723,#28724,#28725,#28726,#28727,#28728,#28729,#28730,
#28731,#28732,#28733,#28734,#28735,#28736,#28737,#28738,#28739,#28740,#28741,
#28742,#28743,#28744,#28745,#28746,#28747,#28748,#28749,#28750,#28751,#28752,
#28753,#28754,#28755,#28756,#28757,#28758,#28759,#28760,#28761,#28762,#28763,
#28764,#28765,#28766,#28767,#28768,#28769,#28770,#28771,#28772,#28773,#28774,
#28775,#28776,#28777,#28778,#28779,#28780,#28781,#28782,#28783,#28784,#28785,
#28786,#28787,#28788,#28789,#28790,#28791,#28792,#28793,#28794,#28795,#28796,
#28797,#28798,#28799,#28800,#28801,#28802,#28803,#28804,#28805,#28806,#28807,
#28808,#28809,#28810,#28811,#28812,#28813,#28814,#28815,#28816,#28817,#28818,
#28819,#28820,#28821,#28822,#28823,#28824,#28825,#28826,#28827,#28828,#28829,
#28830,#28831,#28832,#28833,#28834,#28835,#28836,#28837,#28838,#28839,#28840,
#28841,#28842,#28843,#28844,#28845,#28846,#28847,#28848,#28849,#28850,#28851,
#28852,#28853,#28854,#28855,#28856,#28857,#28858,#28859,#28860,#28861,#28862,
#28863,#28864,#28865,#28866,#28867,#28868,#28869,#28870,#28871,#28872,#28873,
#28874,#28875,#28876,#28877,#28878,#28879,#28880,#28881,#28882,#28883,#28884,
#28885,#28886,#28887,#28888,#28889,#28890,#28891,#28892,#28893,#28894,#28895,
#28896,#28897,#28898,#28899,#28900,#28901,#28902,#28903,#28904,#28905,#28906,
#28907,#28908,#28909,#28910,#28911,#28912,#28913,#28914,#28915,#28916,#28917,
#28918,#28919,#28920,#28921,#28922,#28923,#28924,#28925,#28926,#28927,#28928,
#28929,#28930,#28931,#28932,#28933,#28934,#28935,#28936,#28937,#28938,#28939,
#28940,#28941,#28942,#28943,#28944,#28945,#28946,#28947,#28948,#28949,#28950,
#28951,#28952,#28953,#28954,#28955,#28956,#28957,#28958,#28959,#28960,#28961,
#28962,#28963,#28964,#28965,#28966,#28967,#28968,#28969,#28970,#28971,#28972,
#28973,#28974,#28975,#28976,#28977,#28978,#28979,#28980,#28981,#28982,#28983,
#28984,#28985,#28986,#28987,#28988,#28989,#28990,#28991,#28992,#28993,#28994,
#28995,#28996,#28997,#28998,#28999,#29000,#29001,#29002,#29003,#29004,#29005,
#29006,#29007,#29008,#29009,#29010,#29011,#29012,#29013,#29014,#29015,#29016,
#29017,#29018,#29019,#29020,#29021,#29022,#29023,#29024,#29025,#29026,#29027,
#29028,#29029,#29030,#29031,#29032,#29033,#29034,#29035,#29036,#29037,#29038,
#29039,#29040,#29041,#29042,#29043,#29044,#29045,#29046,#29047,#29048,#29049,
#29050,#29051,#29052,#29053,#29054,#29055,#29056,#29057,#29058,#29059,#29060,
#29061,#29062,#29063,#29064,#29065,#29066,#29067,#29068,#29069,#29070,#29071),
 .UNSPECIFIED.,.F.,.F.,(4,3,3,3,3,3,3,3,3,3,3,3,3,3,3,3,3,3,3,3,3,3,3,3,
3,3,3,3,3,3,3,3,3,3,3,3,3,3,3,3,3,3,3,3,3,3,3,3,3,3,3,3,3,3,3,3,3,3,3,3,
3,3,3,3,3,3,3,3,3,3,3,3,3,3,3,3,3,3,3,3,3,3,3,3,3,3,3,3,3,3,3,3,3,3,3,3,
3,3,3,3,3,3,3,3,3,3,3,3,3,3,3,3,3,3,3,3,3,3,3,3,3,3,3,3,3,3,4),(0.219197959928519,
0.221561939635842,0.222568084891394,0.222573536212963,0.225521953279716,
0.225938209854269,0.225945565409889,0.228899400741101,0.229308334817144,
0.229315162107022,0.232678459780019,0.232683807174909,0.23941870970577,
0.239419709772932,0.246154269068837,0.24615895963152,0.252887867831646,
0.25289920955727,0.256254394695028,0.256269334520146,0.259620875989218,
0.259639459483021,0.273086779141874,0.273119959334522,0.286552662168457,
0.286600459186022,0.300018539495296,0.300080959037523,0.303385007721931,
0.303451084000398,0.306751479243036,0.306821208963274,0.313484421786241,
0.313561458889024,0.326950319411585,0.327041958740525,0.340416230672734,
0.340522458592025,0.347149188045422,0.347262708517776,0.350515662378619,
0.350632833480651,0.353882144673237,0.354002958443526,0.367348212398027,
0.367483458295027,0.380814786959129,0.380963958146528,0.387548398940738,
0.394282341493094,0.394444457998029,0.397649472177266,0.397814582960904,
0.401016888220728,0.401184707923779,0.405374640221065,0.407754831391867,
0.40792495784953,0.410662353985238,0.411126004115685,0.411295082812405,
0.413791286746707,0.414499346528745,0.41466520777528,0.415976012040286,
0.416187126755619,0.416350270256718,0.41739616230529,0.417876132158158,
0.418035332738155,0.419036083859736,0.419567899304777,0.419720395219593,
0.420492219658592,0.421195376093865,0.421264044097592,0.42140545770103,
0.421878321078495,0.422114709919513,0.422247988941749,0.422778375402946,
0.422968274381381,0.423090520182468,0.423396677144126,0.423778766392894,
0.423826452478747,0.423933051423187,0.424179502894481,0.424257716513561,
0.424354317043546,0.424583239235609,0.424690806953789,0.424775582663906,
0.425008747616126,0.425124948394551,0.425196848284265,0.425433747395109,
0.425559819081613,0.425618113904624,0.425936254136417,0.425993896086829,
0.426039379524984,0.426322139644522,0.426426703567751,0.426460645145343,
0.426905273846551,0.427287123039787,0.427303176386062,0.427853616496466,
0.42814235868823,0.428145707626781,0.428662176887248,0.4289882388675,0.428993655368323,
0.429532687076055,0.429830770108219,0.429837872940089,0.430516322774704,
0.430673301348937,0.431009296324422,0.43137348857443,0.431509007896478,
0.431515832589656,0.432713569432477,0.433195104231628,0.434601834369309,
0.434885957552532),.UNSPECIFIED.);
#1116=B_SPLINE_CURVE_WITH_KNOTS('',3,(#29085,#29086,#29087,#29088,#29089,
#29090,#29091,#29092,#29093,#29094,#29095,#29096,#29097,#29098,#29099,#29100,
#29101,#29102,#29103,#29104,#29105,#29106,#29107,#29108,#29109,#29110,#29111,
#29112,#29113,#29114,#29115,#29116,#29117,#29118,#29119,#29120,#29121,#29122,
#29123,#29124,#29125,#29126,#29127,#29128,#29129,#29130,#29131,#29132,#29133,
#29134,#29135,#29136,#29137,#29138,#29139,#29140,#29141,#29142,#29143,#29144,
#29145,#29146,#29147,#29148,#29149,#29150,#29151,#29152,#29153,#29154,#29155,
#29156,#29157,#29158,#29159,#29160,#29161,#29162,#29163,#29164,#29165,#29166,
#29167,#29168,#29169,#29170,#29171,#29172,#29173,#29174,#29175,#29176,#29177,
#29178,#29179,#29180,#29181,#29182,#29183,#29184,#29185,#29186,#29187,#29188,
#29189,#29190,#29191,#29192,#29193,#29194,#29195,#29196,#29197,#29198,#29199,
#29200,#29201,#29202,#29203,#29204,#29205,#29206,#29207,#29208,#29209,#29210,
#29211,#29212,#29213,#29214,#29215,#29216,#29217,#29218,#29219,#29220,#29221,
#29222,#29223,#29224,#29225,#29226,#29227,#29228,#29229,#29230,#29231,#29232,
#29233,#29234,#29235,#29236,#29237,#29238,#29239,#29240,#29241,#29242,#29243,
#29244,#29245,#29246,#29247,#29248,#29249,#29250,#29251,#29252,#29253,#29254,
#29255,#29256,#29257,#29258,#29259,#29260,#29261,#29262,#29263,#29264,#29265,
#29266,#29267,#29268,#29269,#29270,#29271,#29272,#29273,#29274,#29275,#29276,
#29277,#29278,#29279,#29280,#29281,#29282,#29283,#29284,#29285,#29286,#29287,
#29288,#29289,#29290,#29291,#29292,#29293,#29294,#29295,#29296,#29297,#29298,
#29299,#29300,#29301,#29302,#29303,#29304,#29305,#29306,#29307,#29308,#29309,
#29310,#29311,#29312,#29313,#29314,#29315,#29316,#29317,#29318,#29319,#29320,
#29321,#29322,#29323,#29324,#29325,#29326,#29327,#29328,#29329,#29330,#29331,
#29332,#29333,#29334,#29335,#29336,#29337,#29338,#29339,#29340,#29341,#29342,
#29343,#29344,#29345,#29346,#29347,#29348,#29349,#29350,#29351,#29352,#29353,
#29354,#29355),.UNSPECIFIED.,.F.,.F.,(4,3,3,3,3,3,3,3,3,3,3,3,3,3,3,3,3,
3,3,3,3,3,3,3,3,3,3,3,3,3,3,3,3,3,3,3,3,3,3,3,3,3,3,3,3,3,3,3,3,3,3,3,3,
3,3,3,3,3,3,3,3,3,3,3,3,3,3,3,3,3,3,3,3,3,3,3,3,3,3,3,3,3,3,3,3,3,3,3,3,
3,4),(0.0034429235827854,0.00572320515136817,0.00681409602568749,0.00957936021906904,
0.0101852684685896,0.0136633472913732,0.0169276133543937,0.0216348837645216,
0.0236699582401979,0.0263702387236477,0.0290689423761318,0.0304123031260021,
0.0349964377927312,0.0371546480118062,0.0396086289033257,0.042063926447067,
0.0438969928976104,0.0481532478627733,0.0524236025363501,0.0567093502317182,
0.0573816826692188,0.06174126798354,0.0663038202121836,0.0708663724408272,
0.0751777428891207,0.0794798820405295,0.0837649362753547,0.0843510622124355,
0.0886023464618641,0.0910934070982397,0.0952853955230474,0.0978357519840439,
0.102135545828145,0.106445937902228,0.110766418873797,0.111320441755652,
0.115670199879133,0.120237665703197,0.124805131527261,0.129052845127648,
0.13328789796319,0.137501313256485,0.138289821298869,0.14219369664852,0.145032166184673,
0.149378357587458,0.151774511070477,0.156199296918911,0.160729248880498,
0.165259200842086,0.169719242146463,0.174231566380079,0.178743890613694,
0.180619504999544,0.182115063056596,0.185486235499498,0.189107659841198,
0.192228580385302,0.195144301436354,0.195599752828204,0.19805031374221,
0.198970925271106,0.200656511492557,0.201815686763459,0.202342097714009,
0.203704624246645,0.20402768393546,0.205173489201687,0.205713270156911,
0.206440715127883,0.207203427929388,0.207398856378362,0.208142330961523,
0.208241649489087,0.209084442599813,0.209505839155175,0.209927235710538,
0.210348632265901,0.210770028821264,0.211191425376626,0.211612821931989,
0.212239081157345,0.212455615042715,0.21329840815344,0.214011586971214,
0.214141201264166,0.215229565569696,0.215826787485617,0.216979396477024,
0.217512373707068,0.219197959928519),.UNSPECIFIED.);
#1117=B_SPLINE_CURVE_WITH_KNOTS('',3,(#29645,#29646,#29647,#29648,#29649,
#29650,#29651,#29652,#29653,#29654,#29655,#29656,#29657,#29658,#29659,#29660,
#29661,#29662,#29663,#29664,#29665,#29666,#29667,#29668,#29669,#29670,#29671,
#29672,#29673,#29674,#29675,#29676,#29677,#29678,#29679,#29680,#29681,#29682,
#29683,#29684,#29685,#29686,#29687,#29688,#29689,#29690,#29691,#29692,#29693,
#29694,#29695,#29696,#29697,#29698,#29699,#29700,#29701,#29702,#29703,#29704,
#29705,#29706,#29707,#29708,#29709,#29710,#29711,#29712,#29713,#29714,#29715,
#29716,#29717,#29718,#29719,#29720,#29721,#29722,#29723,#29724,#29725,#29726,
#29727,#29728,#29729,#29730,#29731,#29732,#29733,#29734,#29735,#29736,#29737,
#29738,#29739,#29740,#29741,#29742,#29743,#29744,#29745,#29746,#29747,#29748,
#29749,#29750,#29751,#29752,#29753,#29754,#29755,#29756,#29757,#29758,#29759,
#29760,#29761,#29762,#29763,#29764,#29765,#29766,#29767,#29768,#29769,#29770,
#29771,#29772,#29773,#29774,#29775,#29776,#29777,#29778,#29779,#29780,#29781,
#29782,#29783,#29784,#29785,#29786,#29787,#29788,#29789,#29790,#29791,#29792,
#29793,#29794,#29795,#29796,#29797,#29798,#29799,#29800,#29801,#29802,#29803,
#29804,#29805,#29806,#29807,#29808,#29809,#29810,#29811,#29812,#29813,#29814,
#29815,#29816,#29817,#29818,#29819,#29820,#29821,#29822,#29823,#29824,#29825,
#29826,#29827,#29828,#29829,#29830,#29831,#29832,#29833,#29834,#29835,#29836,
#29837,#29838,#29839,#29840,#29841,#29842,#29843,#29844,#29845,#29846,#29847,
#29848,#29849,#29850,#29851,#29852,#29853,#29854,#29855,#29856,#29857,#29858,
#29859,#29860,#29861,#29862,#29863,#29864,#29865,#29866,#29867,#29868,#29869,
#29870,#29871,#29872,#29873,#29874,#29875,#29876,#29877,#29878,#29879,#29880,
#29881,#29882,#29883,#29884,#29885,#29886,#29887,#29888,#29889,#29890,#29891,
#29892,#29893,#29894,#29895,#29896,#29897,#29898,#29899,#29900,#29901,#29902,
#29903,#29904,#29905,#29906,#29907,#29908,#29909,#29910,#29911,#29912,#29913,
#29914,#29915,#29916,#29917,#29918,#29919,#29920,#29921,#29922,#29923,#29924,
#29925,#29926,#29927,#29928,#29929,#29930,#29931,#29932,#29933,#29934,#29935,
#29936,#29937,#29938,#29939,#29940,#29941,#29942,#29943,#29944,#29945,#29946,
#29947,#29948,#29949,#29950,#29951,#29952,#29953,#29954,#29955,#29956,#29957,
#29958,#29959,#29960,#29961,#29962,#29963,#29964,#29965,#29966,#29967,#29968,
#29969,#29970,#29971,#29972,#29973,#29974,#29975,#29976,#29977,#29978,#29979,
#29980,#29981,#29982,#29983,#29984,#29985,#29986,#29987,#29988,#29989,#29990,
#29991,#29992,#29993,#29994,#29995,#29996,#29997,#29998,#29999),
 .UNSPECIFIED.,.F.,.F.,(4,3,3,3,3,3,3,3,3,3,3,3,3,3,3,3,3,3,3,3,3,3,3,3,
3,3,3,3,3,3,3,3,3,3,3,3,3,3,3,3,3,3,3,3,3,3,3,3,3,3,3,3,3,3,3,3,3,3,3,3,
3,3,3,3,3,3,3,3,3,3,3,3,3,3,3,3,3,3,3,3,3,3,3,3,3,3,3,3,3,3,3,3,3,3,3,3,
3,3,3,3,3,3,3,3,3,3,3,3,3,3,3,3,3,3,3,3,3,3,4),(0.00557323536012404,0.00813317970068968,
0.00899310447168613,0.00899708454320929,0.0121711318036108,0.0124129735832482,
0.0124180817258657,0.0155952691298109,0.0158328426948103,0.0158371230923959,
0.0192527118063724,0.0192553994766634,0.0260908370914267,0.0260924500294965,
0.0329251951059827,0.0329321882526206,0.0397587811276712,0.0397719264757448,
0.0431753551494948,0.0431917955873068,0.0465918925264685,0.0466116646988689,
0.0602580243360313,0.0602911411451171,0.0739241399711004,0.0739706175913654,
0.0875902510252554,0.0876500940376136,0.0910067777520482,0.0910699631491756,
0.0944233074266285,0.0944898322607377,0.101256366068591,0.101329570483862,
0.114922493436243,0.11500904693011,0.128588631762366,0.128688523376358,
0.13542170232537,0.135528261599482,0.138838233799944,0.138948130711044,
0.142254772288456,0.142367999822606,0.155921036358478,0.156047476268855,
0.169587707753517,0.169726952715103,0.176421304432259,0.18325516671409,
0.183406429161351,0.186672225782196,0.186826298272913,0.190089514568395,
0.190246167384475,0.194686066878316,0.19692659272522,0.197085905607599,
0.19994345888875,0.200346901177744,0.200505774719161,0.203140343629623,
0.203768953747021,0.203925643830723,0.205275623472084,0.205480868880759,
0.205635578386504,0.206726606049008,0.207193774472377,0.207345512942285,
0.208386484884662,0.208908899872059,0.209055447498066,0.209841495103125,
0.210571007656769,0.210627542708183,0.210765382053847,0.211254417816863,
0.211488962777378,0.211620349331738,0.212183813013997,0.212352708772903,
0.212475316609628,0.212785889588788,0.213193811336146,0.213220178090878,
0.213330283887519,0.213581340987045,0.213655668182996,0.213757767526464,
0.213985258897261,0.214092652619984,0.214185251165409,0.214421594048797,
0.21453045366287,0.214612734804355,0.214839128215605,0.214968872499077,
0.2150402184433,0.215406642448134,0.215753074760998,0.215843362999165,0.21589518572119,
0.21651084508489,0.216712652071532,0.216750152999081,0.217427362517899,
0.217577731954515,0.217605120276971,0.218159809721273,0.218439895499696,
0.218460087554862,0.219300288731891,0.219315054832752,0.220437296311934,
0.221017808849557,0.221024989388533,0.222735034793048,0.224444858500095),
 .UNSPECIFIED.);
#1682=LINE('',#28379,#3255);
#1683=LINE('',#28384,#3256);
#1684=LINE('',#29077,#3257);
#1685=LINE('',#29080,#3258);
#3255=VECTOR('',#21064,14.);
#3256=VECTOR('',#21071,14.);
#3257=VECTOR('',#21080,15.);
#3258=VECTOR('',#21083,15.);
#4646=CYLINDRICAL_SURFACE('',#18738,14.);
#4647=CYLINDRICAL_SURFACE('',#18740,14.);
#4648=CYLINDRICAL_SURFACE('',#18744,15.);
#4649=CYLINDRICAL_SURFACE('',#18746,15.);
#4650=CYLINDRICAL_SURFACE('',#18750,147.404667636179);
#4651=CYLINDRICAL_SURFACE('',#18751,148.404667636179);
#5008=FACE_OUTER_BOUND('',#6079,.T.);
#5009=FACE_OUTER_BOUND('',#6080,.T.);
#5010=FACE_OUTER_BOUND('',#6081,.T.);
#5011=FACE_OUTER_BOUND('',#6082,.T.);
#5012=FACE_OUTER_BOUND('',#6083,.T.);
#5013=FACE_OUTER_BOUND('',#6084,.T.);
#5014=FACE_OUTER_BOUND('',#6085,.T.);
#5015=FACE_OUTER_BOUND('',#6086,.T.);
#5016=FACE_OUTER_BOUND('',#6087,.T.);
#5017=FACE_OUTER_BOUND('',#6089,.T.);
#5018=FACE_OUTER_BOUND('',#6091,.T.);
#5019=FACE_OUTER_BOUND('',#6092,.T.);
#5020=FACE_OUTER_BOUND('',#6093,.T.);
#5021=FACE_OUTER_BOUND('',#6094,.T.);
#6079=EDGE_LOOP('',(#13002,#13003,#13004,#13005,#13006,#13007,#13008,#13009,
#13010,#13011,#13012,#13013));
#6080=EDGE_LOOP('',(#13014,#13015,#13016,#13017,#13018,#13019,#13020,#13021,
#13022,#13023,#13024,#13025));
#6081=EDGE_LOOP('',(#13026,#13027,#13028,#13029,#13030));
#6082=EDGE_LOOP('',(#13031,#13032,#13033,#13034,#13035));
#6083=EDGE_LOOP('',(#13036,#13037,#13038,#13039,#13040));
#6084=EDGE_LOOP('',(#13041,#13042,#13043,#13044,#13045));
#6085=EDGE_LOOP('',(#13046,#13047,#13048,#13049,#13050));
#6086=EDGE_LOOP('',(#13051,#13052,#13053,#13054,#13055));
#6087=EDGE_LOOP('',(#13056));
#6088=EDGE_LOOP('',(#13057));
#6089=EDGE_LOOP('',(#13058));
#6090=EDGE_LOOP('',(#13059));
#6091=EDGE_LOOP('',(#13060,#13061));
#6092=EDGE_LOOP('',(#13062,#13063,#13064,#13065,#13066));
#6093=EDGE_LOOP('',(#13067,#13068));
#6094=EDGE_LOOP('',(#13069,#13070,#13071,#13072,#13073));
#7171=CIRCLE('',#18723,14.);
#7172=CIRCLE('',#18724,208.);
#7173=CIRCLE('',#18725,208.);
#7174=CIRCLE('',#18726,14.);
#7175=CIRCLE('',#18727,14.);
#7176=CIRCLE('',#18728,14.);
#7177=CIRCLE('',#18730,15.);
#7178=CIRCLE('',#18731,15.);
#7179=CIRCLE('',#18732,207.);
#7180=CIRCLE('',#18733,207.);
#7181=CIRCLE('',#18734,15.);
#7182=CIRCLE('',#18735,15.);
#7183=CIRCLE('',#18736,3.99999999999999);
#7184=CIRCLE('',#18737,3.99999999999999);
#7185=CIRCLE('',#18739,14.);
#7186=CIRCLE('',#18741,14.);
#7187=CIRCLE('',#18742,5.);
#7188=CIRCLE('',#18743,5.00000000000001);
#7189=CIRCLE('',#18745,15.);
#7190=CIRCLE('',#18747,15.);
#8000=VERTEX_POINT('',#27161);
#8001=VERTEX_POINT('',#27162);
#8002=VERTEX_POINT('',#27164);
#8003=VERTEX_POINT('',#27166);
#8004=VERTEX_POINT('',#27267);
#8005=VERTEX_POINT('',#27346);
#8006=VERTEX_POINT('',#27348);
#8007=VERTEX_POINT('',#27351);
#8008=VERTEX_POINT('',#27448);
#8009=VERTEX_POINT('',#27449);
#8010=VERTEX_POINT('',#27452);
#8011=VERTEX_POINT('',#27454);
#8012=VERTEX_POINT('',#27531);
#8013=VERTEX_POINT('',#27629);
#8014=VERTEX_POINT('',#27631);
#8015=VERTEX_POINT('',#27634);
#8016=VERTEX_POINT('',#28102);
#8017=VERTEX_POINT('',#28103);
#8018=VERTEX_POINT('',#28378);
#8019=VERTEX_POINT('',#28382);
#8020=VERTEX_POINT('',#28691);
#8021=VERTEX_POINT('',#28692);
#8022=VERTEX_POINT('',#29075);
#8023=VERTEX_POINT('',#29079);
#9881=EDGE_CURVE('',#8000,#8001,#7171,.T.);
#9882=EDGE_CURVE('',#8000,#8002,#7172,.T.);
#9883=EDGE_CURVE('',#8003,#8002,#1106,.T.);
#9884=EDGE_CURVE('',#8004,#8003,#1107,.T.);
#9885=EDGE_CURVE('',#8004,#8005,#7173,.T.);
#9886=EDGE_CURVE('',#8005,#8006,#7174,.T.);
#9887=EDGE_CURVE('',#8006,#8005,#7175,.T.);
#9888=EDGE_CURVE('',#8007,#8004,#1108,.T.);
#9889=EDGE_CURVE('',#8002,#8007,#1109,.T.);
#9890=EDGE_CURVE('',#8001,#8000,#7176,.T.);
#9891=EDGE_CURVE('',#8008,#8009,#7177,.T.);
#9892=EDGE_CURVE('',#8009,#8008,#7178,.T.);
#9893=EDGE_CURVE('',#8009,#8010,#7179,.T.);
#9894=EDGE_CURVE('',#8010,#8011,#1110,.T.);
#9895=EDGE_CURVE('',#8011,#8012,#1111,.T.);
#9896=EDGE_CURVE('',#8012,#8013,#7180,.T.);
#9897=EDGE_CURVE('',#8013,#8014,#7181,.T.);
#9898=EDGE_CURVE('',#8014,#8013,#7182,.T.);
#9899=EDGE_CURVE('',#8012,#8015,#1112,.T.);
#9900=EDGE_CURVE('',#8015,#8010,#1113,.T.);
#9901=EDGE_CURVE('',#8016,#8017,#1114,.T.);
#9902=EDGE_CURVE('',#8017,#8003,#7183,.T.);
#9903=EDGE_CURVE('',#8016,#8007,#7184,.T.);
#9904=EDGE_CURVE('',#8006,#8018,#1682,.T.);
#9905=EDGE_CURVE('',#8018,#8018,#7185,.T.);
#9906=EDGE_CURVE('',#8019,#8019,#7186,.T.);
#9907=EDGE_CURVE('',#8019,#8001,#1683,.T.);
#9908=EDGE_CURVE('',#8020,#8021,#1115,.T.);
#9909=EDGE_CURVE('',#8020,#8011,#7187,.T.);
#9910=EDGE_CURVE('',#8021,#8015,#7188,.T.);
#9911=EDGE_CURVE('',#8022,#8022,#7189,.T.);
#9912=EDGE_CURVE('',#8022,#8008,#1684,.T.);
#9913=EDGE_CURVE('',#8014,#8023,#1685,.T.);
#9914=EDGE_CURVE('',#8023,#8023,#7190,.T.);
#9915=EDGE_CURVE('',#8021,#8020,#1116,.T.);
#9916=EDGE_CURVE('',#8017,#8016,#1117,.T.);
#13002=ORIENTED_EDGE('',*,*,#9881,.F.);
#13003=ORIENTED_EDGE('',*,*,#9882,.T.);
#13004=ORIENTED_EDGE('',*,*,#9883,.F.);
#13005=ORIENTED_EDGE('',*,*,#9884,.F.);
#13006=ORIENTED_EDGE('',*,*,#9885,.T.);
#13007=ORIENTED_EDGE('',*,*,#9886,.T.);
#13008=ORIENTED_EDGE('',*,*,#9887,.T.);
#13009=ORIENTED_EDGE('',*,*,#9885,.F.);
#13010=ORIENTED_EDGE('',*,*,#9888,.F.);
#13011=ORIENTED_EDGE('',*,*,#9889,.F.);
#13012=ORIENTED_EDGE('',*,*,#9882,.F.);
#13013=ORIENTED_EDGE('',*,*,#9890,.F.);
#13014=ORIENTED_EDGE('',*,*,#9891,.F.);
#13015=ORIENTED_EDGE('',*,*,#9892,.F.);
#13016=ORIENTED_EDGE('',*,*,#9893,.T.);
#13017=ORIENTED_EDGE('',*,*,#9894,.T.);
#13018=ORIENTED_EDGE('',*,*,#9895,.T.);
#13019=ORIENTED_EDGE('',*,*,#9896,.T.);
#13020=ORIENTED_EDGE('',*,*,#9897,.T.);
#13021=ORIENTED_EDGE('',*,*,#9898,.T.);
#13022=ORIENTED_EDGE('',*,*,#9896,.F.);
#13023=ORIENTED_EDGE('',*,*,#9899,.T.);
#13024=ORIENTED_EDGE('',*,*,#9900,.T.);
#13025=ORIENTED_EDGE('',*,*,#9893,.F.);
#13026=ORIENTED_EDGE('',*,*,#9901,.T.);
#13027=ORIENTED_EDGE('',*,*,#9902,.T.);
#13028=ORIENTED_EDGE('',*,*,#9883,.T.);
#13029=ORIENTED_EDGE('',*,*,#9889,.T.);
#13030=ORIENTED_EDGE('',*,*,#9903,.F.);
#13031=ORIENTED_EDGE('',*,*,#9887,.F.);
#13032=ORIENTED_EDGE('',*,*,#9904,.T.);
#13033=ORIENTED_EDGE('',*,*,#9905,.T.);
#13034=ORIENTED_EDGE('',*,*,#9904,.F.);
#13035=ORIENTED_EDGE('',*,*,#9886,.F.);
#13036=ORIENTED_EDGE('',*,*,#9906,.F.);
#13037=ORIENTED_EDGE('',*,*,#9907,.T.);
#13038=ORIENTED_EDGE('',*,*,#9890,.T.);
#13039=ORIENTED_EDGE('',*,*,#9881,.T.);
#13040=ORIENTED_EDGE('',*,*,#9907,.F.);
#13041=ORIENTED_EDGE('',*,*,#9908,.F.);
#13042=ORIENTED_EDGE('',*,*,#9909,.T.);
#13043=ORIENTED_EDGE('',*,*,#9894,.F.);
#13044=ORIENTED_EDGE('',*,*,#9900,.F.);
#13045=ORIENTED_EDGE('',*,*,#9910,.F.);
#13046=ORIENTED_EDGE('',*,*,#9911,.F.);
#13047=ORIENTED_EDGE('',*,*,#9912,.T.);
#13048=ORIENTED_EDGE('',*,*,#9891,.T.);
#13049=ORIENTED_EDGE('',*,*,#9892,.T.);
#13050=ORIENTED_EDGE('',*,*,#9912,.F.);
#13051=ORIENTED_EDGE('',*,*,#9897,.F.);
#13052=ORIENTED_EDGE('',*,*,#9898,.F.);
#13053=ORIENTED_EDGE('',*,*,#9913,.T.);
#13054=ORIENTED_EDGE('',*,*,#9914,.T.);
#13055=ORIENTED_EDGE('',*,*,#9913,.F.);
#13056=ORIENTED_EDGE('',*,*,#9911,.T.);
#13057=ORIENTED_EDGE('',*,*,#9905,.F.);
#13058=ORIENTED_EDGE('',*,*,#9914,.F.);
#13059=ORIENTED_EDGE('',*,*,#9906,.T.);
#13060=ORIENTED_EDGE('',*,*,#9915,.T.);
#13061=ORIENTED_EDGE('',*,*,#9908,.T.);
#13062=ORIENTED_EDGE('',*,*,#9909,.F.);
#13063=ORIENTED_EDGE('',*,*,#9915,.F.);
#13064=ORIENTED_EDGE('',*,*,#9910,.T.);
#13065=ORIENTED_EDGE('',*,*,#9899,.F.);
#13066=ORIENTED_EDGE('',*,*,#9895,.F.);
#13067=ORIENTED_EDGE('',*,*,#9901,.F.);
#13068=ORIENTED_EDGE('',*,*,#9916,.F.);
#13069=ORIENTED_EDGE('',*,*,#9902,.F.);
#13070=ORIENTED_EDGE('',*,*,#9916,.T.);
#13071=ORIENTED_EDGE('',*,*,#9903,.T.);
#13072=ORIENTED_EDGE('',*,*,#9888,.T.);
#13073=ORIENTED_EDGE('',*,*,#9884,.T.);
#17254=TOROIDAL_SURFACE('',#18722,222.,14.);
#17255=TOROIDAL_SURFACE('',#18729,222.,15.);
#17452=ADVANCED_FACE('',(#5008),#17254,.F.);
#17453=ADVANCED_FACE('',(#5009),#17255,.T.);
#17454=ADVANCED_FACE('',(#5010),#184,.F.);
#17455=ADVANCED_FACE('',(#5011),#4646,.F.);
#17456=ADVANCED_FACE('',(#5012),#4647,.F.);
#17457=ADVANCED_FACE('',(#5013),#185,.T.);
#17458=ADVANCED_FACE('',(#5014),#4648,.T.);
#17459=ADVANCED_FACE('',(#5015),#4649,.T.);
#17460=ADVANCED_FACE('',(#5016,#954),#389,.T.);
#17461=ADVANCED_FACE('',(#5017,#955),#390,.F.);
#17462=ADVANCED_FACE('',(#5018),#4650,.F.);
#17463=ADVANCED_FACE('',(#5019),#186,.T.);
#17464=ADVANCED_FACE('',(#5020),#4651,.T.);
#17465=ADVANCED_FACE('',(#5021),#187,.F.);
#18261=CLOSED_SHELL('',(#17452,#17453,#17454,#17455,#17456,#17457,#17458,
#17459,#17460,#17461,#17462,#17463,#17464,#17465));
#18721=AXIS2_PLACEMENT_3D('',#27159,#21028,#21029);
#18722=AXIS2_PLACEMENT_3D('',#27160,#21030,#21031);
#18723=AXIS2_PLACEMENT_3D('',#27163,#21032,#21033);
#18724=AXIS2_PLACEMENT_3D('',#27165,#21034,#21035);
#18725=AXIS2_PLACEMENT_3D('',#27347,#21036,#21037);
#18726=AXIS2_PLACEMENT_3D('',#27349,#21038,#21039);
#18727=AXIS2_PLACEMENT_3D('',#27350,#21040,#21041);
#18728=AXIS2_PLACEMENT_3D('',#27446,#21042,#21043);
#18729=AXIS2_PLACEMENT_3D('',#27447,#21044,#21045);
#18730=AXIS2_PLACEMENT_3D('',#27450,#21046,#21047);
#18731=AXIS2_PLACEMENT_3D('',#27451,#21048,#21049);
#18732=AXIS2_PLACEMENT_3D('',#27453,#21050,#21051);
#18733=AXIS2_PLACEMENT_3D('',#27630,#21052,#21053);
#18734=AXIS2_PLACEMENT_3D('',#27632,#21054,#21055);
#18735=AXIS2_PLACEMENT_3D('',#27633,#21056,#21057);
#18736=AXIS2_PLACEMENT_3D('',#28375,#21058,#21059);
#18737=AXIS2_PLACEMENT_3D('',#28376,#21060,#21061);
#18738=AXIS2_PLACEMENT_3D('',#28377,#21062,#21063);
#18739=AXIS2_PLACEMENT_3D('',#28380,#21065,#21066);
#18740=AXIS2_PLACEMENT_3D('',#28381,#21067,#21068);
#18741=AXIS2_PLACEMENT_3D('',#28383,#21069,#21070);
#18742=AXIS2_PLACEMENT_3D('',#29072,#21072,#21073);
#18743=AXIS2_PLACEMENT_3D('',#29073,#21074,#21075);
#18744=AXIS2_PLACEMENT_3D('',#29074,#21076,#21077);
#18745=AXIS2_PLACEMENT_3D('',#29076,#21078,#21079);
#18746=AXIS2_PLACEMENT_3D('',#29078,#21081,#21082);
#18747=AXIS2_PLACEMENT_3D('',#29081,#21084,#21085);
#18748=AXIS2_PLACEMENT_3D('',#29082,#21086,#21087);
#18749=AXIS2_PLACEMENT_3D('',#29083,#21088,#21089);
#18750=AXIS2_PLACEMENT_3D('',#29084,#21090,#21091);
#18751=AXIS2_PLACEMENT_3D('',#29644,#21092,#21093);
#21028=DIRECTION('axis',(0.,0.,1.));
#21029=DIRECTION('refdir',(1.,0.,0.));
#21030=DIRECTION('center_axis',(0.,0.,1.));
#21031=DIRECTION('ref_axis',(-1.,1.22464679914735E-16,0.));
#21032=DIRECTION('center_axis',(-1.,6.12323399573677E-17,0.));
#21033=DIRECTION('ref_axis',(6.12323399573677E-17,1.,0.));
#21034=DIRECTION('center_axis',(0.,0.,1.));
#21035=DIRECTION('ref_axis',(-1.,1.22464679914735E-16,0.));
#21036=DIRECTION('center_axis',(0.,0.,1.));
#21037=DIRECTION('ref_axis',(-1.,1.22464679914735E-16,0.));
#21038=DIRECTION('center_axis',(1.,0.,0.));
#21039=DIRECTION('ref_axis',(0.,0.,-1.));
#21040=DIRECTION('center_axis',(1.,0.,0.));
#21041=DIRECTION('ref_axis',(0.,0.,-1.));
#21042=DIRECTION('center_axis',(-1.,6.12323399573677E-17,0.));
#21043=DIRECTION('ref_axis',(6.12323399573677E-17,1.,0.));
#21044=DIRECTION('center_axis',(0.,0.,1.));
#21045=DIRECTION('ref_axis',(-1.,1.22464679914735E-16,0.));
#21046=DIRECTION('center_axis',(1.,2.55123084520842E-16,0.));
#21047=DIRECTION('ref_axis',(-2.55123084520842E-16,1.,0.));
#21048=DIRECTION('center_axis',(1.,2.55123084520842E-16,0.));
#21049=DIRECTION('ref_axis',(-2.55123084520842E-16,1.,0.));
#21050=DIRECTION('center_axis',(0.,0.,-1.));
#21051=DIRECTION('ref_axis',(-1.,1.22464679914735E-16,0.));
#21052=DIRECTION('center_axis',(0.,0.,-1.));
#21053=DIRECTION('ref_axis',(-1.,1.22464679914735E-16,0.));
#21054=DIRECTION('center_axis',(-1.,-4.38820104392945E-16,0.));
#21055=DIRECTION('ref_axis',(4.38820104392945E-16,-1.,0.));
#21056=DIRECTION('center_axis',(-1.,-4.38820104392945E-16,0.));
#21057=DIRECTION('ref_axis',(4.38820104392945E-16,-1.,0.));
#21058=DIRECTION('center_axis',(-0.582556010419622,-0.750905958805901,0.311076736117899));
#21059=DIRECTION('ref_axis',(0.790107291694676,-0.612968569839355,-3.50006659356662E-16));
#21060=DIRECTION('center_axis',(-0.582614729034438,0.755300040476885,-0.300136512886627));
#21061=DIRECTION('ref_axis',(-0.791805223116158,-0.610773680380852,1.37374746571133E-16));
#21062=DIRECTION('center_axis',(1.,0.,0.));
#21063=DIRECTION('ref_axis',(0.,0.,-1.));
#21064=DIRECTION('',(1.,0.,0.));
#21065=DIRECTION('center_axis',(1.,4.38820104392945E-16,0.));
#21066=DIRECTION('ref_axis',(-4.38820104392945E-16,1.,0.));
#21067=DIRECTION('center_axis',(-1.,0.,0.));
#21068=DIRECTION('ref_axis',(0.,0.,1.));
#21069=DIRECTION('center_axis',(-1.,-4.38820104392945E-16,0.));
#21070=DIRECTION('ref_axis',(4.38820104392945E-16,-1.,0.));
#21071=DIRECTION('',(-1.,0.,0.));
#21072=DIRECTION('center_axis',(-0.582556010419622,-0.750905958805901,0.311076736117899));
#21073=DIRECTION('ref_axis',(0.790107291694676,-0.612968569839355,-4.40287716331881E-16));
#21074=DIRECTION('center_axis',(-0.582614729034438,0.755300040476885,-0.300136512886627));
#21075=DIRECTION('ref_axis',(-0.791805223116158,-0.610773680380852,2.90913046502425E-16));
#21076=DIRECTION('center_axis',(1.,0.,0.));
#21077=DIRECTION('ref_axis',(0.,0.,-1.));
#21078=DIRECTION('center_axis',(1.,4.38820104392945E-16,0.));
#21079=DIRECTION('ref_axis',(-4.38820104392945E-16,1.,0.));
#21080=DIRECTION('',(-1.,0.,0.));
#21081=DIRECTION('center_axis',(-1.,0.,0.));
#21082=DIRECTION('ref_axis',(0.,0.,1.));
#21083=DIRECTION('',(1.,0.,0.));
#21084=DIRECTION('center_axis',(-1.,-4.38820104392945E-16,0.));
#21085=DIRECTION('ref_axis',(4.38820104392945E-16,-1.,0.));
#21086=DIRECTION('center_axis',(1.,4.38820104392945E-16,0.));
#21087=DIRECTION('ref_axis',(-4.38820104392945E-16,1.,0.));
#21088=DIRECTION('center_axis',(-1.,-4.38820104392945E-16,0.));
#21089=DIRECTION('ref_axis',(4.38820104392945E-16,-1.,0.));
#21090=DIRECTION('center_axis',(0.,0.,1.));
#21091=DIRECTION('ref_axis',(-0.999999999995711,2.92869692484868E-6,0.));
#21092=DIRECTION('center_axis',(0.,0.,1.));
#21093=DIRECTION('ref_axis',(-0.999999999989654,4.54879961062145E-6,0.));
#27159=CARTESIAN_POINT('',(0.,0.,0.));
#27160=CARTESIAN_POINT('Origin',(0.,0.,0.));
#27161=CARTESIAN_POINT('',(1.27363267111325E-14,208.,-1.71450551880629E-15));
#27162=CARTESIAN_POINT('',(0.,222.,-14.));
#27163=CARTESIAN_POINT('Origin',(1.35935794705356E-14,222.,0.));
#27164=CARTESIAN_POINT('',(-183.924299418847,97.1383141879995,-2.45234074816238E-11));
#27165=CARTESIAN_POINT('Origin',(0.,0.,-1.71450551880629E-15));
#27166=CARTESIAN_POINT('',(-188.965207680627,91.9372213898726,7.4447346109596));
#27167=CARTESIAN_POINT('Ctrl Pts',(-188.965207680626,91.9372213898729,7.44473461095943));
#27168=CARTESIAN_POINT('Ctrl Pts',(-188.777281065684,92.1417492337039,7.31811198115176));
#27169=CARTESIAN_POINT('Ctrl Pts',(-188.589786144602,92.3445422191641,7.18727696952707));
#27170=CARTESIAN_POINT('Ctrl Pts',(-188.402949359252,92.5454067376809,7.05154332610887));
#27171=CARTESIAN_POINT('Ctrl Pts',(-188.216112573901,92.7462712561977,6.91580968269067));
#27172=CARTESIAN_POINT('Ctrl Pts',(-188.029934009438,92.9452072423305,6.77517683974821));
#27173=CARTESIAN_POINT('Ctrl Pts',(-187.84463499754,93.142030410138,6.62901215662966));
#27174=CARTESIAN_POINT('Ctrl Pts',(-187.685431029225,93.3111356258137,6.50343135972319));
#27175=CARTESIAN_POINT('Ctrl Pts',(-187.526731368968,93.478830345021,6.37369884055212));
#27176=CARTESIAN_POINT('Ctrl Pts',(-187.368931721517,93.644742838303,6.23917845532948));
#27177=CARTESIAN_POINT('Ctrl Pts',(-187.358712366937,93.6554875936023,6.23046670256522));
#27178=CARTESIAN_POINT('Ctrl Pts',(-187.348496782088,93.6662248798462,6.22173488584732));
#27179=CARTESIAN_POINT('Ctrl Pts',(-187.338285072337,93.6769545984829,6.21298283941028));
#27180=CARTESIAN_POINT('Ctrl Pts',(-187.204548187013,93.8174755480478,6.09836232440827));
#27181=CARTESIAN_POINT('Ctrl Pts',(-187.071431813471,93.9567739444096,5.98026061216412));
#27182=CARTESIAN_POINT('Ctrl Pts',(-186.939063717966,94.0947139001685,5.85818571601648));
#27183=CARTESIAN_POINT('Ctrl Pts',(-186.869499901573,94.167205913588,5.79403131665466));
#27184=CARTESIAN_POINT('Ctrl Pts',(-186.79969674014,94.2397787170827,5.72835556874943));
#27185=CARTESIAN_POINT('Ctrl Pts',(-186.730077654463,94.311986609344,5.66143525552039));
#27186=CARTESIAN_POINT('Ctrl Pts',(-186.667223476599,94.3771780386651,5.60101760956244));
#27187=CARTESIAN_POINT('Ctrl Pts',(-186.604587356584,94.4420013140829,5.53968086297713));
#27188=CARTESIAN_POINT('Ctrl Pts',(-186.542485785002,94.50613245851,5.47761211877966));
#27189=CARTESIAN_POINT('Ctrl Pts',(-186.436000166469,94.6160981873572,5.37118278939107));
#27190=CARTESIAN_POINT('Ctrl Pts',(-186.330692100467,94.7244995729387,5.26228082287464));
#27191=CARTESIAN_POINT('Ctrl Pts',(-186.226759940933,94.831157452253,5.15054882323236));
#27192=CARTESIAN_POINT('Ctrl Pts',(-186.125678797888,94.9348895444588,5.04188180150126));
#27193=CARTESIAN_POINT('Ctrl Pts',(-186.02589914915,95.0369724528684,4.93053778166716));
#27194=CARTESIAN_POINT('Ctrl Pts',(-185.927591324053,95.1372549667413,4.81623371046665));
#27195=CARTESIAN_POINT('Ctrl Pts',(-185.878492805196,95.1873397173047,4.75914608199233));
#27196=CARTESIAN_POINT('Ctrl Pts',(-185.829761217654,95.2369756002562,4.70132084032866));
#27197=CARTESIAN_POINT('Ctrl Pts',(-185.781416555225,95.2861451237541,4.64272728542119));
#27198=CARTESIAN_POINT('Ctrl Pts',(-185.737559874666,95.3307500910229,4.58957314820614));
#27199=CARTESIAN_POINT('Ctrl Pts',(-185.694016468188,95.3749718553161,4.53577438997125));
#27200=CARTESIAN_POINT('Ctrl Pts',(-185.650807802727,95.41879168514,4.4813195101232));
#27201=CARTESIAN_POINT('Ctrl Pts',(-185.574087130878,95.4965975314552,4.38463022516696));
#27202=CARTESIAN_POINT('Ctrl Pts',(-185.498348272351,95.5732099457179,4.28567472753969));
#27203=CARTESIAN_POINT('Ctrl Pts',(-185.424001069689,95.6482394066019,4.18453965879523));
#27204=CARTESIAN_POINT('Ctrl Pts',(-185.352087703078,95.7208126969739,4.08671535585732));
#27205=CARTESIAN_POINT('Ctrl Pts',(-185.281476519291,95.7919048404079,3.98685192836821));
#27206=CARTESIAN_POINT('Ctrl Pts',(-185.212508038807,95.8611936177919,3.88505147091736));
#27207=CARTESIAN_POINT('Ctrl Pts',(-185.188395255985,95.8854183829225,3.84945996151216));
#27208=CARTESIAN_POINT('Ctrl Pts',(-185.164482979243,95.9094230017288,3.81363189217638));
#27209=CARTESIAN_POINT('Ctrl Pts',(-185.140784795543,95.9331946623266,3.77757231362429));
#27210=CARTESIAN_POINT('Ctrl Pts',(-185.121628056577,95.9524107973109,3.74842307829493));
#27211=CARTESIAN_POINT('Ctrl Pts',(-185.102604574441,95.9714814439119,3.71911920337178));
#27212=CARTESIAN_POINT('Ctrl Pts',(-185.083719917007,95.9904016355523,3.68965406509349));
#27213=CARTESIAN_POINT('Ctrl Pts',(-185.024451423954,96.0497816508219,3.59717929559146));
#27214=CARTESIAN_POINT('Ctrl Pts',(-184.966549837208,96.1076881079189,3.50312319977729));
#27215=CARTESIAN_POINT('Ctrl Pts',(-184.91017752504,96.1639721188239,3.40730682859391));
#27216=CARTESIAN_POINT('Ctrl Pts',(-184.854918825039,96.219144261918,3.31338327096742));
#27217=CARTESIAN_POINT('Ctrl Pts',(-184.801129614601,96.2727574049647,3.21776823030466));
#27218=CARTESIAN_POINT('Ctrl Pts',(-184.748944154795,96.3246902126642,3.12033555929367));
#27219=CARTESIAN_POINT('Ctrl Pts',(-184.722937793693,96.3505706658611,3.07178047834085));
#27220=CARTESIAN_POINT('Ctrl Pts',(-184.697329423299,96.3760341107952,3.02277466583946));
#27221=CARTESIAN_POINT('Ctrl Pts',(-184.672133835317,96.4010673582064,2.97330663101595));
#27222=CARTESIAN_POINT('Ctrl Pts',(-184.627607521379,96.4453067795653,2.88588540274296));
#27223=CARTESIAN_POINT('Ctrl Pts',(-184.58424172121,96.4883286304064,2.79669596755631));
#27224=CARTESIAN_POINT('Ctrl Pts',(-184.54235398425,96.5298308010085,2.70593977270456));
#27225=CARTESIAN_POINT('Ctrl Pts',(-184.526333540261,96.5457037807351,2.67122902818081));
#27226=CARTESIAN_POINT('Ctrl Pts',(-184.510528921791,96.561354839112,2.63628916907188));
#27227=CARTESIAN_POINT('Ctrl Pts',(-184.49495645186,96.5767684840588,2.60113170275939));
#27228=CARTESIAN_POINT('Ctrl Pts',(-184.457448604398,96.6138937856985,2.51645143756278));
#27229=CARTESIAN_POINT('Ctrl Pts',(-184.42119837209,96.6497332749268,2.43030849578046));
#27230=CARTESIAN_POINT('Ctrl Pts',(-184.386467350968,96.6840359323964,2.34293783062457));
#27231=CARTESIAN_POINT('Ctrl Pts',(-184.352937166828,96.7171525637043,2.25858803621967));
#27232=CARTESIAN_POINT('Ctrl Pts',(-184.32082314254,96.7488366313688,2.17309415060979));
#27233=CARTESIAN_POINT('Ctrl Pts',(-184.290328389036,96.7788942509748,2.08668618679845));
#27234=CARTESIAN_POINT('Ctrl Pts',(-184.283436100126,96.7856877408207,2.06715664212894));
#27235=CARTESIAN_POINT('Ctrl Pts',(-184.27662638795,96.7923982854362,2.04758047426811));
#27236=CARTESIAN_POINT('Ctrl Pts',(-184.269901344592,96.7990238955975,2.02796046082246));
#27237=CARTESIAN_POINT('Ctrl Pts',(-184.26623686533,96.8026341936638,2.01726950634743));
#27238=CARTESIAN_POINT('Ctrl Pts',(-184.262597332157,96.8062194864247,2.00656547941313));
#27239=CARTESIAN_POINT('Ctrl Pts',(-184.258983022864,96.8097795163212,1.99584840652776));
#27240=CARTESIAN_POINT('Ctrl Pts',(-184.223537518536,96.8446927030049,1.89074615255131));
#27241=CARTESIAN_POINT('Ctrl Pts',(-184.190473176187,96.8772201529816,1.78424485552327));
#27242=CARTESIAN_POINT('Ctrl Pts',(-184.159960059398,96.9072126758638,1.67612419944574));
#27243=CARTESIAN_POINT('Ctrl Pts',(-184.143137275991,96.9237484404584,1.61651408516027));
#27244=CARTESIAN_POINT('Ctrl Pts',(-184.127089415644,96.9395141816105,1.55641233920697));
#27245=CARTESIAN_POINT('Ctrl Pts',(-184.111841067988,96.9544884398172,1.49578619414718));
#27246=CARTESIAN_POINT('Ctrl Pts',(-184.10013259563,96.9659864520781,1.44923429490751));
#27247=CARTESIAN_POINT('Ctrl Pts',(-184.088901899494,96.97701152717,1.40233382499999));
#27248=CARTESIAN_POINT('Ctrl Pts',(-184.078180757733,96.9875336813599,1.35519738700399));
#27249=CARTESIAN_POINT('Ctrl Pts',(-184.058107442441,97.0072344299651,1.26694329964282));
#27250=CARTESIAN_POINT('Ctrl Pts',(-184.039793616161,97.0251959100348,1.17773537467592));
#27251=CARTESIAN_POINT('Ctrl Pts',(-184.023436891388,97.0412305639008,1.08817980520529));
#27252=CARTESIAN_POINT('Ctrl Pts',(-184.013337630761,97.0511309657662,1.03288480885195));
#27253=CARTESIAN_POINT('Ctrl Pts',(-184.003984328087,97.060296937738,0.977456098654038));
#27254=CARTESIAN_POINT('Ctrl Pts',(-183.995422776363,97.06868494987,0.922026700139618));
#27255=CARTESIAN_POINT('Ctrl Pts',(-183.976848898345,97.0868823420241,0.801775264428186));
#27256=CARTESIAN_POINT('Ctrl Pts',(-183.961821282879,97.1015955688319,0.68091917253188));
#27257=CARTESIAN_POINT('Ctrl Pts',(-183.950437303463,97.1127380434133,0.559199366684126));
#27258=CARTESIAN_POINT('Ctrl Pts',(-183.943134370342,97.1198860488431,0.481114931601442));
#27259=CARTESIAN_POINT('Ctrl Pts',(-183.93733152959,97.1255639515528,0.402674791403003));
#27260=CARTESIAN_POINT('Ctrl Pts',(-183.9330622763,97.1297411343775,0.32380729739441));
#27261=CARTESIAN_POINT('Ctrl Pts',(-183.927831946245,97.1348586674432,0.227185477057826));
#27262=CARTESIAN_POINT('Ctrl Pts',(-183.924970282477,97.1376584995943,0.129411875784403));
#27263=CARTESIAN_POINT('Ctrl Pts',(-183.924458161665,97.1381595218518,0.0316528433418993));
#27264=CARTESIAN_POINT('Ctrl Pts',(-183.924402886243,97.138213599358,0.0211012867892161));
#27265=CARTESIAN_POINT('Ctrl Pts',(-183.924375001864,97.138240877262,0.0105498589472018));
#27266=CARTESIAN_POINT('Ctrl Pts',(-183.924374498502,97.1382413655954,-7.00888014293355E-10));
#27267=CARTESIAN_POINT('',(-183.924299418846,-97.1383141879995,1.6286382377323E-15));
#27268=CARTESIAN_POINT('Ctrl Pts',(-183.924299418846,-97.1383141879995,
1.6286382377323E-15));
#27269=CARTESIAN_POINT('Ctrl Pts',(-183.924299418847,-97.1383141879996,
0.289606573667191));
#27270=CARTESIAN_POINT('Ctrl Pts',(-183.945294598411,-97.1177882275971,
0.576128192439725));
#27271=CARTESIAN_POINT('Ctrl Pts',(-184.026954906122,-97.0378030821182,
1.14333145788899));
#27272=CARTESIAN_POINT('Ctrl Pts',(-184.087299204572,-96.9786517847449,
1.42056425530318));
#27273=CARTESIAN_POINT('Ctrl Pts',(-184.239213583142,-96.8293094810531,
1.95495869016732));
#27274=CARTESIAN_POINT('Ctrl Pts',(-184.331762894336,-96.7381490066639,
2.21530983652599));
#27275=CARTESIAN_POINT('Ctrl Pts',(-184.539595228575,-96.5326824648098,
2.71171918629039));
#27276=CARTESIAN_POINT('Ctrl Pts',(-184.654706063204,-96.4185488213364,
2.94816573920908));
#27277=CARTESIAN_POINT('Ctrl Pts',(-185.02647179182,-96.0483938637497,3.62930814728168));
#27278=CARTESIAN_POINT('Ctrl Pts',(-185.311549180074,-95.7625411976457,
4.04843931623329));
#27279=CARTESIAN_POINT('Ctrl Pts',(-185.908081548002,-95.1582117642484,
4.81028372456617));
#27280=CARTESIAN_POINT('Ctrl Pts',(-186.221658835681,-94.8376773560741,
5.15691217997208));
#27281=CARTESIAN_POINT('Ctrl Pts',(-186.868145715832,-94.1697219232036,
5.80304524490739));
#27282=CARTESIAN_POINT('Ctrl Pts',(-187.201193142186,-93.8221709116559,
6.10227777090564));
#27283=CARTESIAN_POINT('Ctrl Pts',(-187.880549907623,-93.1052140686194,
6.66488432085835));
#27284=CARTESIAN_POINT('Ctrl Pts',(-188.22814505543,-92.7344219550961,6.92900726524237));
#27285=CARTESIAN_POINT('Ctrl Pts',(-189.275208253741,-91.6044438981369,
7.67158459471431));
#27286=CARTESIAN_POINT('Ctrl Pts',(-189.976354544114,-90.8305882749372,
8.10040126241789));
#27287=CARTESIAN_POINT('Ctrl Pts',(-191.374588317242,-89.250261707686,8.87382214052879));
#27288=CARTESIAN_POINT('Ctrl Pts',(-192.071836977406,-88.4436449005057,
9.21763122303672));
#27289=CARTESIAN_POINT('Ctrl Pts',(-193.457278361193,-86.8015935109936,
9.84360712907318));
#27290=CARTESIAN_POINT('Ctrl Pts',(-194.145522657778,-85.9661135276441,
10.1255231834183));
#27291=CARTESIAN_POINT('Ctrl Pts',(-196.19191597214,-83.4197910447744,10.8995122536796));
#27292=CARTESIAN_POINT('Ctrl Pts',(-197.531515647658,-81.6692498423691,
11.3208437569989));
#27293=CARTESIAN_POINT('Ctrl Pts',(-199.492190335423,-78.9710560946796,
11.8586418616589));
#27294=CARTESIAN_POINT('Ctrl Pts',(-200.138798925329,-78.0578863331849,
12.0220836807334));
#27295=CARTESIAN_POINT('Ctrl Pts',(-201.40602210199,-76.2205466037287,12.3199232325791));
#27296=CARTESIAN_POINT('Ctrl Pts',(-202.027379911037,-75.2954459129312,
12.4545571141892));
#27297=CARTESIAN_POINT('Ctrl Pts',(-203.854832722202,-72.5012481746631,
12.8226747946999));
#27298=CARTESIAN_POINT('Ctrl Pts',(-205.024317580872,-70.6132750985836,
13.0206893865685));
#27299=CARTESIAN_POINT('Ctrl Pts',(-208.387244631561,-64.8761223846278,
13.5122485336218));
#27300=CARTESIAN_POINT('Ctrl Pts',(-210.435425840902,-60.9539161091157,
13.7050519148717));
#27301=CARTESIAN_POINT('Ctrl Pts',(-214.144176955874,-52.9203842766436,
13.9447223410129));
#27302=CARTESIAN_POINT('Ctrl Pts',(-215.804813106923,-48.8090196665873,
13.9900872820394));
#27303=CARTESIAN_POINT('Ctrl Pts',(-217.998369105242,-42.4995152895031,
14.0027740092237));
#27304=CARTESIAN_POINT('Ctrl Pts',(-218.679912382467,-40.3725573743037,
13.9975347191773));
#27305=CARTESIAN_POINT('Ctrl Pts',(-219.62616267774,-37.1459345955272,13.980864955456));
#27306=CARTESIAN_POINT('Ctrl Pts',(-219.929225739207,-36.0631092234961,
13.9738214451819));
#27307=CARTESIAN_POINT('Ctrl Pts',(-220.508095214681,-33.8911509216661,
13.9576271630892));
#27308=CARTESIAN_POINT('Ctrl Pts',(-220.783424005549,-32.8039498686341,
13.9484949198543));
#27309=CARTESIAN_POINT('Ctrl Pts',(-222.090385807589,-27.3619003043185,
13.8996044768986));
#27310=CARTESIAN_POINT('Ctrl Pts',(-222.913500587235,-22.9889613912764,
13.8509457895095));
#27311=CARTESIAN_POINT('Ctrl Pts',(-224.127738137291,-14.2054494124102,
13.7709601634318));
#27312=CARTESIAN_POINT('Ctrl Pts',(-224.518828150004,-9.79487372996352,
13.7395801077819));
#27313=CARTESIAN_POINT('Ctrl Pts',(-224.869105640044,-0.936019490422407,
13.7117102244513));
#27314=CARTESIAN_POINT('Ctrl Pts',(-224.828321321409,3.51225676594121,13.7152551483673));
#27315=CARTESIAN_POINT('Ctrl Pts',(-224.499599127585,9.09684225070298,13.7409136885715));
#27316=CARTESIAN_POINT('Ctrl Pts',(-224.4199349447,10.2149739885714,13.7470594015732));
#27317=CARTESIAN_POINT('Ctrl Pts',(-224.23243573416,12.4536946433225,13.7611695346538));
#27318=CARTESIAN_POINT('Ctrl Pts',(-224.124563005179,13.5740681295282,13.7691356336449));
#27319=CARTESIAN_POINT('Ctrl Pts',(-223.76071604259,16.9182868017048,13.7951450599868));
#27320=CARTESIAN_POINT('Ctrl Pts',(-223.464013321503,19.1321332304902,13.8153704223117));
#27321=CARTESIAN_POINT('Ctrl Pts',(-222.415051088304,25.7277907019174,13.8795349289317));
#27322=CARTESIAN_POINT('Ctrl Pts',(-221.504313463055,30.0638296946454,13.9274520583673));
#27323=CARTESIAN_POINT('Ctrl Pts',(-219.269264018172,38.6163649455757,13.9942669977442));
#27324=CARTESIAN_POINT('Ctrl Pts',(-217.944936174541,42.8328570669653,14.0133729245824));
#27325=CARTESIAN_POINT('Ctrl Pts',(-214.88002904003,51.1453899765955,13.9654070644487));
#27326=CARTESIAN_POINT('Ctrl Pts',(-213.13949100334,55.2414444523707,13.8990836182993));
#27327=CARTESIAN_POINT('Ctrl Pts',(-210.694370828089,60.283416978766,13.7075079551512));
#27328=CARTESIAN_POINT('Ctrl Pts',(-210.191194888016,61.2891398827893,13.663578611472));
#27329=CARTESIAN_POINT('Ctrl Pts',(-209.16065556682,63.2865110306788,13.5629787339324));
#27330=CARTESIAN_POINT('Ctrl Pts',(-208.633964828839,64.2769408168412,13.5063869810004));
#27331=CARTESIAN_POINT('Ctrl Pts',(-207.020159630544,67.2234096152245,13.3148819803906));
#27332=CARTESIAN_POINT('Ctrl Pts',(-205.899309096341,69.1546564288455,13.1584578298572));
#27333=CARTESIAN_POINT('Ctrl Pts',(-203.570426573057,72.9501257617516,12.7687139843163));
#27334=CARTESIAN_POINT('Ctrl Pts',(-202.362373093814,74.8143635854865,12.5356047498722));
#27335=CARTESIAN_POINT('Ctrl Pts',(-199.862178770943,78.4738596816999,11.9639786153397));
#27336=CARTESIAN_POINT('Ctrl Pts',(-198.569984776825,80.2691602211054,11.6260140633101));
#27337=CARTESIAN_POINT('Ctrl Pts',(-196.57195550953,82.9075286142192,11.0039793996147));
#27338=CARTESIAN_POINT('Ctrl Pts',(-195.89600311974,83.7778708332067,10.7772677458374));
#27339=CARTESIAN_POINT('Ctrl Pts',(-194.525119525015,85.4994949310966,10.2748858952649));
#27340=CARTESIAN_POINT('Ctrl Pts',(-193.83201420713,86.3483748013007,9.99984001499434));
#27341=CARTESIAN_POINT('Ctrl Pts',(-192.443022672674,88.0089491897228,9.39284720135033));
#27342=CARTESIAN_POINT('Ctrl Pts',(-191.745822424016,88.8222836276672,9.06062243030275));
#27343=CARTESIAN_POINT('Ctrl Pts',(-190.352288451153,90.4105500302893,8.31897581534296));
#27344=CARTESIAN_POINT('Ctrl Pts',(-189.655811580761,91.1856103065845,7.91005498091941));
#27345=CARTESIAN_POINT('Ctrl Pts',(-188.965207680627,91.9372213898726,7.4447346109596));
#27346=CARTESIAN_POINT('',(-3.15824218834415E-14,-208.,-1.71450551880629E-15));
#27347=CARTESIAN_POINT('Origin',(0.,0.,-1.71450551880629E-15));
#27348=CARTESIAN_POINT('',(-3.15824218834415E-14,-222.,14.));
#27349=CARTESIAN_POINT('Origin',(-3.15824218834415E-14,-222.,0.));
#27350=CARTESIAN_POINT('Origin',(-3.15824218834415E-14,-222.,0.));
#27351=CARTESIAN_POINT('',(-189.252344883447,-91.6237366354615,-7.63473361656836));
#27352=CARTESIAN_POINT('Ctrl Pts',(-189.252344883447,-91.6237366354615,
-7.63473361656836));
#27353=CARTESIAN_POINT('Ctrl Pts',(-188.666509085829,-92.2653391382624,
-7.2539887318565));
#27354=CARTESIAN_POINT('Ctrl Pts',(-188.089380051022,-92.8849778109279,
-6.83875146569526));
#27355=CARTESIAN_POINT('Ctrl Pts',(-186.968116025761,-94.0679928081637,
-5.90831038164945));
#27356=CARTESIAN_POINT('Ctrl Pts',(-186.423262692469,-94.6320391895917,
-5.39465052751624));
#27357=CARTESIAN_POINT('Ctrl Pts',(-185.655376248049,-95.4148977911641,
-4.49846237685947));
#27358=CARTESIAN_POINT('Ctrl Pts',(-185.406583998279,-95.6663955704661,
-4.17665287330735));
#27359=CARTESIAN_POINT('Ctrl Pts',(-184.940925516141,-96.1338625850361,
-3.47817276299474));
#27360=CARTESIAN_POINT('Ctrl Pts',(-184.726546490054,-96.3473475582936,
-3.10569066952788));
#27361=CARTESIAN_POINT('Ctrl Pts',(-184.354363966567,-96.7160922094891,
-2.29793911795022));
#27362=CARTESIAN_POINT('Ctrl Pts',(-184.201053959324,-96.8669273884385,
-1.87245077917943));
#27363=CARTESIAN_POINT('Ctrl Pts',(-184.038570146028,-97.0264280245017,
-1.19046756850576));
#27364=CARTESIAN_POINT('Ctrl Pts',(-183.995900054248,-97.0682280802022,
-0.955005769387058));
#27365=CARTESIAN_POINT('Ctrl Pts',(-183.9389953264,-97.1239440434863,-0.481662656210902));
#27366=CARTESIAN_POINT('Ctrl Pts',(-183.924299418846,-97.1383141879995,
-0.241197781359841));
#27367=CARTESIAN_POINT('Ctrl Pts',(-183.924299418846,-97.1383141879995,
1.6286382377323E-15));
#27368=CARTESIAN_POINT('Ctrl Pts',(-183.924299418847,97.1383141879995,-2.45234074816238E-11));
#27369=CARTESIAN_POINT('Ctrl Pts',(-183.924299418848,97.1383141879982,-0.289293301043451));
#27370=CARTESIAN_POINT('Ctrl Pts',(-183.945246216988,97.1178352743025,-0.574831380827163));
#27371=CARTESIAN_POINT('Ctrl Pts',(-184.026168974811,97.0385732297218,-1.13882338953088));
#27372=CARTESIAN_POINT('Ctrl Pts',(-184.086353500478,96.9795792606563,-1.41641997278048));
#27373=CARTESIAN_POINT('Ctrl Pts',(-184.237290286536,96.8312023888215,-1.94899521951201));
#27374=CARTESIAN_POINT('Ctrl Pts',(-184.328773586646,96.7410972488276,-2.20734178770506));
#27375=CARTESIAN_POINT('Ctrl Pts',(-184.536045978299,96.5361981324799,-2.70404415625005));
#27376=CARTESIAN_POINT('Ctrl Pts',(-184.650675626616,96.4225494185532,-2.94010876392827));
#27377=CARTESIAN_POINT('Ctrl Pts',(-184.897041418233,96.1772753531742,-3.3928151445005));
#27378=CARTESIAN_POINT('Ctrl Pts',(-185.028806857472,96.0456213657732,-3.60942484353172));
#27379=CARTESIAN_POINT('Ctrl Pts',(-185.306190021303,95.7671972032446,-4.02660699512156));
#27380=CARTESIAN_POINT('Ctrl Pts',(-185.452123042776,95.620101727754,-4.22741942202966));
#27381=CARTESIAN_POINT('Ctrl Pts',(-185.899177016858,95.1672867203483,-4.79996460051786));
#27382=CARTESIAN_POINT('Ctrl Pts',(-186.211874696161,94.8477060015223,-5.14633171366901));
#27383=CARTESIAN_POINT('Ctrl Pts',(-187.177253870719,93.8505055701753,-6.11354637057988));
#27384=CARTESIAN_POINT('Ctrl Pts',(-187.856598791335,93.134972043538,-6.66377670847504));
#27385=CARTESIAN_POINT('Ctrl Pts',(-188.899602703674,92.0099908210452,-7.40602386987046));
#27386=CARTESIAN_POINT('Ctrl Pts',(-189.251093155014,91.6265899532315,-7.63854891641251));
#27387=CARTESIAN_POINT('Ctrl Pts',(-189.951287505344,90.8538465649765,-8.07489972933164));
#27388=CARTESIAN_POINT('Ctrl Pts',(-190.301206659029,90.4632019265966,-8.27956354245871));
#27389=CARTESIAN_POINT('Ctrl Pts',(-191.348977896207,89.2796407946467,-8.86065506893184));
#27390=CARTESIAN_POINT('Ctrl Pts',(-192.044773452492,88.4751580400445,-9.20456317412189));
#27391=CARTESIAN_POINT('Ctrl Pts',(-193.426080088475,86.8391100951027,-9.83031641121458));
#27392=CARTESIAN_POINT('Ctrl Pts',(-194.111639716675,86.0075020766135,-10.1118965188247));
#27393=CARTESIAN_POINT('Ctrl Pts',(-196.148613709987,83.4751543078266,-10.8846927099913));
#27394=CARTESIAN_POINT('Ctrl Pts',(-197.480133504116,81.7370594032411,-11.305004133147));
#27395=CARTESIAN_POINT('Ctrl Pts',(-199.427277956411,79.061736809832,-11.8416503383128));
#27396=CARTESIAN_POINT('Ctrl Pts',(-200.068037672566,78.1585401083653,-12.0045286228002));
#27397=CARTESIAN_POINT('Ctrl Pts',(-201.331792808165,76.3299028888316,-12.3033005273701));
#27398=CARTESIAN_POINT('Ctrl Pts',(-201.955766490901,75.4029324575626,-12.4393616147252));
#27399=CARTESIAN_POINT('Ctrl Pts',(-203.789380826525,72.6050223527821,-12.8109057765609));
#27400=CARTESIAN_POINT('Ctrl Pts',(-204.962444257487,70.7149876206329,-13.0106557132063));
#27401=CARTESIAN_POINT('Ctrl Pts',(-208.334885204917,64.97284066522,-13.5064989325318));
#27402=CARTESIAN_POINT('Ctrl Pts',(-210.387791961828,61.0488867819828,-13.7009628268141));
#27403=CARTESIAN_POINT('Ctrl Pts',(-214.104196849767,53.0150029671012,-13.9431260054544));
#27404=CARTESIAN_POINT('Ctrl Pts',(-215.767750838602,48.9050361592617,-13.989284646881));
#27405=CARTESIAN_POINT('Ctrl Pts',(-217.965171860694,42.6001126302614,-14.002865883644));
#27406=CARTESIAN_POINT('Ctrl Pts',(-218.647916793637,40.4750969194813,-13.9978706752266));
#27407=CARTESIAN_POINT('Ctrl Pts',(-219.595939962548,37.2520377674546,-13.9815031003));
#27408=CARTESIAN_POINT('Ctrl Pts',(-219.899368743631,36.171187315868,-13.9745517151795));
#27409=CARTESIAN_POINT('Ctrl Pts',(-220.477440402961,34.0097240519904,-13.9585793089129));
#27410=CARTESIAN_POINT('Ctrl Pts',(-220.752532941888,32.9276497263176,-13.9495525121151));
#27411=CARTESIAN_POINT('Ctrl Pts',(-222.059068051356,27.510631885896,-13.9011404780045));
#27412=CARTESIAN_POINT('Ctrl Pts',(-222.884242784183,23.1557959145204,-13.8526891852329));
#27413=CARTESIAN_POINT('Ctrl Pts',(-224.106142919279,14.404638181653,-13.772559117181));
#27414=CARTESIAN_POINT('Ctrl Pts',(-224.502841203057,10.0083140242484,-13.7408321408321));
#27415=CARTESIAN_POINT('Ctrl Pts',(-224.866867117856,1.17400800753462,-13.711907328236));
#27416=CARTESIAN_POINT('Ctrl Pts',(-224.83422743905,-3.26397087488992,-13.7147485874252));
#27417=CARTESIAN_POINT('Ctrl Pts',(-224.453183725159,-9.95315272494675,
-13.7445574981991));
#27418=CARTESIAN_POINT('Ctrl Pts',(-224.269875506322,-12.1940962642215,
-13.7586615908191));
#27419=CARTESIAN_POINT('Ctrl Pts',(-223.795577148681,-16.6370922798083,
-13.7927293726463));
#27420=CARTESIAN_POINT('Ctrl Pts',(-223.504633439409,-18.8435115295463,
-13.8126877638542));
#27421=CARTESIAN_POINT('Ctrl Pts',(-222.473806565301,-25.4184761287494,
-13.8762990186828));
#27422=CARTESIAN_POINT('Ctrl Pts',(-221.576298994197,-29.7428330952291,
-13.9241751615609));
#27423=CARTESIAN_POINT('Ctrl Pts',(-219.369230163102,-38.2759802604658,
-13.992319185983));
#27424=CARTESIAN_POINT('Ctrl Pts',(-218.059656539427,-42.4847672627358,
-14.0127887068107));
#27425=CARTESIAN_POINT('Ctrl Pts',(-215.025133999908,-50.7857678762348,
-13.9698621357405));
#27426=CARTESIAN_POINT('Ctrl Pts',(-213.300229963115,-54.8779950418535,
-13.907191527293));
#27427=CARTESIAN_POINT('Ctrl Pts',(-210.874797903038,-59.9176309101772,
-13.7225218764077));
#27428=CARTESIAN_POINT('Ctrl Pts',(-210.375538180112,-60.9230450669806,
-13.6800873300562));
#27429=CARTESIAN_POINT('Ctrl Pts',(-209.354416026681,-62.9170286488566,
-13.5829151958296));
#27430=CARTESIAN_POINT('Ctrl Pts',(-208.832334628704,-63.9061429936345,
-13.5281755289986));
#27431=CARTESIAN_POINT('Ctrl Pts',(-207.231970951578,-66.8497997256187,
-13.3426795325515));
#27432=CARTESIAN_POINT('Ctrl Pts',(-206.119569880797,-68.7806813058041,
-13.1908611905979));
#27433=CARTESIAN_POINT('Ctrl Pts',(-203.806019801973,-72.5784926687438,
-12.8117980747563));
#27434=CARTESIAN_POINT('Ctrl Pts',(-202.604853069669,-74.4454352778335,
-12.5847577915574));
#27435=CARTESIAN_POINT('Ctrl Pts',(-200.116163488173,-78.1135836520715,
-12.0271908520484));
#27436=CARTESIAN_POINT('Ctrl Pts',(-198.82859706036,-79.9148244022689,-11.6971965579858));
#27437=CARTESIAN_POINT('Ctrl Pts',(-196.835024756913,-82.5648480465928,
-11.0892859689757));
#27438=CARTESIAN_POINT('Ctrl Pts',(-196.161413841412,-83.4377758103841,
-10.8679626155705));
#27439=CARTESIAN_POINT('Ctrl Pts',(-194.803373031953,-85.1545718645404,
-10.3812253616273));
#27440=CARTESIAN_POINT('Ctrl Pts',(-194.11814612319,-85.999497126127,-10.1156542867041));
#27441=CARTESIAN_POINT('Ctrl Pts',(-192.738313170377,-87.6603590181507,
-9.52788750796532));
#27442=CARTESIAN_POINT('Ctrl Pts',(-192.043668081395,-88.4763296708027,
-9.20586973247695));
#27443=CARTESIAN_POINT('Ctrl Pts',(-190.649625487509,-90.0758715417795,
-8.48578531610911));
#27444=CARTESIAN_POINT('Ctrl Pts',(-189.950117761389,-90.8595415714283,
-8.0882283586907));
#27445=CARTESIAN_POINT('Ctrl Pts',(-189.252344883447,-91.6237366354615,
-7.63473361656836));
#27446=CARTESIAN_POINT('Origin',(1.35935794705356E-14,222.,0.));
#27447=CARTESIAN_POINT('Origin',(0.,0.,0.));
#27448=CARTESIAN_POINT('',(-3.15824218834415E-14,-222.,15.));
#27449=CARTESIAN_POINT('',(-3.15824218834415E-14,-207.,-1.83697019872103E-15));
#27450=CARTESIAN_POINT('Origin',(-2.77555756156289E-14,-222.,0.));
#27451=CARTESIAN_POINT('Origin',(-2.77555756156289E-14,-222.,0.));
#27452=CARTESIAN_POINT('',(-183.040047979333,-96.6713030620957,1.55769866206538E-14));
#27453=CARTESIAN_POINT('Origin',(0.,0.,-1.83697019872103E-15));
#27454=CARTESIAN_POINT('',(-188.203666712899,91.5667089479117,7.97650136887543));
#27455=CARTESIAN_POINT('Ctrl Pts',(-183.040047979333,-96.6713030620957,
1.55769866197491E-14));
#27456=CARTESIAN_POINT('Ctrl Pts',(-183.040047979333,-96.6713030620956,
0.291148679290596));
#27457=CARTESIAN_POINT('Ctrl Pts',(-183.058980950331,-96.6535943415814,
0.57974868924173));
#27458=CARTESIAN_POINT('Ctrl Pts',(-183.132993285616,-96.5842492219133,
1.15207487751939));
#27459=CARTESIAN_POINT('Ctrl Pts',(-183.188070480362,-96.5326105208468,
1.43412348751035));
#27460=CARTESIAN_POINT('Ctrl Pts',(-183.327967184294,-96.4010948894287,
1.98002353439478));
#27461=CARTESIAN_POINT('Ctrl Pts',(-183.413460182539,-96.3205813016289,
2.24681133290275));
#27462=CARTESIAN_POINT('Ctrl Pts',(-183.608674914206,-96.1360952072225,
2.76184779141642));
#27463=CARTESIAN_POINT('Ctrl Pts',(-183.717592481392,-96.0328819217764,
3.00851618547335));
#27464=CARTESIAN_POINT('Ctrl Pts',(-183.953720315568,-95.8082188834415,
3.4840703792612));
#27465=CARTESIAN_POINT('Ctrl Pts',(-184.080951141305,-95.6867496989865,
3.71293669895085));
#27466=CARTESIAN_POINT('Ctrl Pts',(-184.350664529886,-95.4280873250007,
4.15559630117501));
#27467=CARTESIAN_POINT('Ctrl Pts',(-184.493074751668,-95.2909557075865,
4.36905997833143));
#27468=CARTESIAN_POINT('Ctrl Pts',(-184.931498282134,-94.8667492919688,
4.97954692467032));
#27469=CARTESIAN_POINT('Ctrl Pts',(-185.241141223251,-94.5645177651879,
5.35155104444554));
#27470=CARTESIAN_POINT('Ctrl Pts',(-186.203958736528,-93.6146152438495,
6.39425281757349));
#27471=CARTESIAN_POINT('Ctrl Pts',(-186.891302371369,-92.9233052227938,
6.99367622818273));
#27472=CARTESIAN_POINT('Ctrl Pts',(-188.305681714773,-91.4656918334382,
8.07241329266994));
#27473=CARTESIAN_POINT('Ctrl Pts',(-189.018430897681,-90.7143285017377,
8.53970972029528));
#27474=CARTESIAN_POINT('Ctrl Pts',(-190.442802070271,-89.1760731637858,
9.38285699584151));
#27475=CARTESIAN_POINT('Ctrl Pts',(-191.15461822974,-88.3890133117134,9.7578302902465));
#27476=CARTESIAN_POINT('Ctrl Pts',(-192.571192569202,-86.7836262630972,
10.4408468314537));
#27477=CARTESIAN_POINT('Ctrl Pts',(-193.27601245978,-85.96524723729,10.748615183262));
#27478=CARTESIAN_POINT('Ctrl Pts',(-195.374252691012,-83.4669421359547,
11.5939771576598));
#27479=CARTESIAN_POINT('Ctrl Pts',(-196.751203470348,-81.7440535365057,
12.0547297956035));
#27480=CARTESIAN_POINT('Ctrl Pts',(-198.769971299121,-79.0815725360579,
12.6433844340074));
#27481=CARTESIAN_POINT('Ctrl Pts',(-199.436591021777,-78.1790237365388,
12.8224654289728));
#27482=CARTESIAN_POINT('Ctrl Pts',(-200.744763817792,-76.3598416721392,
13.1491235542598));
#27483=CARTESIAN_POINT('Ctrl Pts',(-201.386303874719,-75.4433717087901,
13.2967666638446));
#27484=CARTESIAN_POINT('Ctrl Pts',(-203.273408069987,-72.6737796512646,
13.7004868908735));
#27485=CARTESIAN_POINT('Ctrl Pts',(-204.481466008945,-70.8004978383475,
13.9177067702817));
#27486=CARTESIAN_POINT('Ctrl Pts',(-207.956458983342,-65.1026091973039,
14.4573854330589));
#27487=CARTESIAN_POINT('Ctrl Pts',(-210.074493786179,-61.2001921411133,
14.6697866179376));
#27488=CARTESIAN_POINT('Ctrl Pts',(-213.912886037181,-53.1943214976126,
14.9353299175372));
#27489=CARTESIAN_POINT('Ctrl Pts',(-215.633323467389,-49.0908222055926,
14.986792054574));
#27490=CARTESIAN_POINT('Ctrl Pts',(-217.908396227818,-42.7841937443938,
15.0032413379716));
#27491=CARTESIAN_POINT('Ctrl Pts',(-218.615742309528,-40.6567017058131,
14.998335228712));
#27492=CARTESIAN_POINT('Ctrl Pts',(-219.926088227278,-36.350417240132,14.9755428583751));
#27493=CARTESIAN_POINT('Ctrl Pts',(-220.529800921946,-34.1674257024326,
14.9575922154785));
#27494=CARTESIAN_POINT('Ctrl Pts',(-222.161510126542,-27.6207361803836,
14.8952029196392));
#27495=CARTESIAN_POINT('Ctrl Pts',(-223.018675922415,-23.2357106926463,
14.8428468498203));
#27496=CARTESIAN_POINT('Ctrl Pts',(-224.286108963103,-14.4256282001768,
14.7563556073774));
#27497=CARTESIAN_POINT('Ctrl Pts',(-224.696337066657,-10.0005680076165,
14.7221538153805));
#27498=CARTESIAN_POINT('Ctrl Pts',(-225.070163176114,-1.11035032097217,
14.6912120318798));
#27499=CARTESIAN_POINT('Ctrl Pts',(-225.033793040228,3.35480449941421,14.6945093265208));
#27500=CARTESIAN_POINT('Ctrl Pts',(-224.700737496435,8.96206207694743,14.721618144576));
#27501=CARTESIAN_POINT('Ctrl Pts',(-224.619710847452,10.0848072650507,14.7281381219928));
#27502=CARTESIAN_POINT('Ctrl Pts',(-224.428465136887,12.3329162515791,14.7431531378288));
#27503=CARTESIAN_POINT('Ctrl Pts',(-224.318164098119,13.458479623482,14.7516532939685));
#27504=CARTESIAN_POINT('Ctrl Pts',(-223.945632319424,16.8171559006165,14.7794486414301));
#27505=CARTESIAN_POINT('Ctrl Pts',(-223.641247849546,19.0396172614184,14.8011160303732));
#27506=CARTESIAN_POINT('Ctrl Pts',(-222.563939303659,25.6581889778629,14.8699597930253));
#27507=CARTESIAN_POINT('Ctrl Pts',(-221.627271804797,30.0056107522321,14.9215038566953));
#27508=CARTESIAN_POINT('Ctrl Pts',(-219.327317476923,38.5734928326465,14.9935819020374));
#27509=CARTESIAN_POINT('Ctrl Pts',(-217.964011313114,42.793947973277,15.0143464053309));
#27510=CARTESIAN_POINT('Ctrl Pts',(-214.807994247347,51.1069121038375,14.9632933929592));
#27511=CARTESIAN_POINT('Ctrl Pts',(-213.015330352922,55.1994371694619,14.8923013616224));
#27512=CARTESIAN_POINT('Ctrl Pts',(-210.496052823544,60.2319818480121,14.6864216598738));
#27513=CARTESIAN_POINT('Ctrl Pts',(-209.977518875153,61.2356634382941,14.6391865829707));
#27514=CARTESIAN_POINT('Ctrl Pts',(-208.915699033734,63.2279335470269,14.530991204538));
#27515=CARTESIAN_POINT('Ctrl Pts',(-208.373138206947,64.2152547465443,14.4701199370589));
#27516=CARTESIAN_POINT('Ctrl Pts',(-206.711108280302,67.1507229882156,14.2641249010502));
#27517=CARTESIAN_POINT('Ctrl Pts',(-205.55728638811,69.0724061150207,14.0958534464656));
#27518=CARTESIAN_POINT('Ctrl Pts',(-203.161251585093,72.8442174373689,13.6766605958867));
#27519=CARTESIAN_POINT('Ctrl Pts',(-201.919013597683,74.6943624357747,13.4259631930999));
#27520=CARTESIAN_POINT('Ctrl Pts',(-199.349782492321,78.3209577812108,12.8114190642419));
#27521=CARTESIAN_POINT('Ctrl Pts',(-198.022727586167,80.0974546194972,12.4481581938624));
#27522=CARTESIAN_POINT('Ctrl Pts',(-195.97252063722,82.7037994050085,11.7799394449392));
#27523=CARTESIAN_POINT('Ctrl Pts',(-195.279197353805,83.562828999768,11.5364478286467));
#27524=CARTESIAN_POINT('Ctrl Pts',(-193.873779899557,85.2604683721014,10.9970720898174));
#27525=CARTESIAN_POINT('Ctrl Pts',(-193.164004359316,86.0961634161304,10.7020151751908));
#27526=CARTESIAN_POINT('Ctrl Pts',(-191.743919945876,87.7276352163228,10.0519934684016));
#27527=CARTESIAN_POINT('Ctrl Pts',(-191.032198859638,88.5251060018795,9.69668774260903));
#27528=CARTESIAN_POINT('Ctrl Pts',(-189.612385303067,90.078853967896,8.9054582820669));
#27529=CARTESIAN_POINT('Ctrl Pts',(-188.904144762275,90.8352574843552,8.47000883192016));
#27530=CARTESIAN_POINT('Ctrl Pts',(-188.203666712899,91.5667089479117,7.97650136887543));
#27531=CARTESIAN_POINT('',(-183.040047979333,96.6713030620956,-1.78040965343628E-11));
#27532=CARTESIAN_POINT('Ctrl Pts',(-188.203666712899,91.5667089479117,7.97650136887544));
#27533=CARTESIAN_POINT('Ctrl Pts',(-188.021076801371,91.7573725356387,7.84786138637183));
#27534=CARTESIAN_POINT('Ctrl Pts',(-187.839014153582,91.9463367031238,7.7152484090642));
#27535=CARTESIAN_POINT('Ctrl Pts',(-187.657688363759,92.1334355047595,7.57806657321992));
#27536=CARTESIAN_POINT('Ctrl Pts',(-187.482614389677,92.3140834466786,7.44561454200802));
#27537=CARTESIAN_POINT('Ctrl Pts',(-187.308227372814,92.4929924341846,7.30890311629443));
#27538=CARTESIAN_POINT('Ctrl Pts',(-187.134710929371,92.6700205956967,7.16744440176363));
#27539=CARTESIAN_POINT('Ctrl Pts',(-187.108293925377,92.6969722410681,7.14590802542574));
#27540=CARTESIAN_POINT('Ctrl Pts',(-187.081897089628,92.7238803062719,7.1242617107976));
#27541=CARTESIAN_POINT('Ctrl Pts',(-187.055521058621,92.7507443066074,7.10250384250346));
#27542=CARTESIAN_POINT('Ctrl Pts',(-186.902111764284,92.9069917470796,6.97595488521369));
#27543=CARTESIAN_POINT('Ctrl Pts',(-186.749275961903,93.0618767690438,6.84556443583174));
#27544=CARTESIAN_POINT('Ctrl Pts',(-186.597357972257,93.2150934975638,6.71079465634692));
#27545=CARTESIAN_POINT('Ctrl Pts',(-186.562877573727,93.2498686672017,6.68020633881195));
#27546=CARTESIAN_POINT('Ctrl Pts',(-186.528444397317,93.2845579577452,6.64939261767227));
#27547=CARTESIAN_POINT('Ctrl Pts',(-186.494062363408,93.3191579039876,6.61834755243621));
#27548=CARTESIAN_POINT('Ctrl Pts',(-186.387663841254,93.4262307768882,6.52227560189259));
#27549=CARTESIAN_POINT('Ctrl Pts',(-186.281628729357,93.5325860908707,6.42388081224351));
#27550=CARTESIAN_POINT('Ctrl Pts',(-186.176231882927,93.6379436507861,6.32312127204413));
#27551=CARTESIAN_POINT('Ctrl Pts',(-186.088224400876,93.7259183281816,6.23898598976658));
#27552=CARTESIAN_POINT('Ctrl Pts',(-186.000661983538,93.8131974648858,6.15320249997137));
#27553=CARTESIAN_POINT('Ctrl Pts',(-185.913702242406,93.8996252320157,6.06577333665428));
#27554=CARTESIAN_POINT('Ctrl Pts',(-185.830659834658,93.98215962995,5.98228265309385));
#27555=CARTESIAN_POINT('Ctrl Pts',(-185.748282632558,94.0638023049231,5.89745987433741));
#27556=CARTESIAN_POINT('Ctrl Pts',(-185.666724552854,94.1444112466403,5.81120124899772));
#27557=CARTESIAN_POINT('Ctrl Pts',(-185.565754072301,94.2442066760027,5.70441140200803));
#27558=CARTESIAN_POINT('Ctrl Pts',(-185.465966572545,94.3425454523725,5.59540453025664));
#27559=CARTESIAN_POINT('Ctrl Pts',(-185.36752368835,94.4392774100917,5.4838933269904));
#27560=CARTESIAN_POINT('Ctrl Pts',(-185.271466218412,94.5336654117913,5.37508420235797));
#27561=CARTESIAN_POINT('Ctrl Pts',(-185.176689032625,94.6265235208791,5.26389056210744));
#27562=CARTESIAN_POINT('Ctrl Pts',(-185.083333271035,94.7177251966252,5.15009214619747));
#27563=CARTESIAN_POINT('Ctrl Pts',(-185.017242203712,94.7822912822002,5.06952873330148));
#27564=CARTESIAN_POINT('Ctrl Pts',(-184.95186335678,94.8460274452087,4.98766078741659));
#27565=CARTESIAN_POINT('Ctrl Pts',(-184.88724379259,94.9088928760068,4.9044251869639));
#27566=CARTESIAN_POINT('Ctrl Pts',(-184.860768537757,94.9346494455754,4.87032276363793));
#27567=CARTESIAN_POINT('Ctrl Pts',(-184.834419684901,94.9602607323629,4.83598937607995));
#27568=CARTESIAN_POINT('Ctrl Pts',(-184.80820176871,94.9857229573254,4.80142347587037));
#27569=CARTESIAN_POINT('Ctrl Pts',(-184.732754718691,95.0589953618257,4.70195351101801));
#27570=CARTESIAN_POINT('Ctrl Pts',(-184.658322875617,95.1310996942388,4.60036233156195));
#27571=CARTESIAN_POINT('Ctrl Pts',(-184.585276389778,95.2016996031477,4.49675562307688));
#27572=CARTESIAN_POINT('Ctrl Pts',(-184.514231589108,95.2703648701778,4.39598803832812));
#27573=CARTESIAN_POINT('Ctrl Pts',(-184.444497389723,95.3376069258162,4.29331394586699));
#27574=CARTESIAN_POINT('Ctrl Pts',(-184.376383333509,95.4031461308148,4.18885474060621));
#27575=CARTESIAN_POINT('Ctrl Pts',(-184.345867348177,95.4325085492294,4.14205565459065));
#27576=CARTESIAN_POINT('Ctrl Pts',(-184.315676117797,95.4615295939936,4.09489859062733));
#27577=CARTESIAN_POINT('Ctrl Pts',(-184.285835279432,95.4901862208126,4.04739604433558));
#27578=CARTESIAN_POINT('Ctrl Pts',(-184.250347078743,95.5242660985678,3.9909036671654));
#27579=CARTESIAN_POINT('Ctrl Pts',(-184.215332259082,95.5578521322308,3.93391060486237));
#27580=CARTESIAN_POINT('Ctrl Pts',(-184.180823297309,95.5909168803663,3.87638066206044));
#27581=CARTESIAN_POINT('Ctrl Pts',(-184.122135163681,95.6471488924924,3.77854158498635));
#27582=CARTESIAN_POINT('Ctrl Pts',(-184.06492944055,95.7018658475249,3.67919720543105));
#27583=CARTESIAN_POINT('Ctrl Pts',(-184.009332974402,95.7549582674443,3.57817784229945));
#27584=CARTESIAN_POINT('Ctrl Pts',(-183.954092701837,95.80771053662,3.47780568665149));
#27585=CARTESIAN_POINT('Ctrl Pts',(-183.900441148331,95.8588590170415,3.37577991412729));
#27586=CARTESIAN_POINT('Ctrl Pts',(-183.848484126247,95.908314252787,3.27197868131283));
#27587=CARTESIAN_POINT('Ctrl Pts',(-183.834151916205,95.921956351544,3.24334537994841));
#27588=CARTESIAN_POINT('Ctrl Pts',(-183.819948535722,95.9354697139894,3.21457724453099));
#27589=CARTESIAN_POINT('Ctrl Pts',(-183.805875952186,95.9488527047503,3.18567232341047));
#27590=CARTESIAN_POINT('Ctrl Pts',(-183.760917696567,95.9916078902521,3.09332859497882));
#27591=CARTESIAN_POINT('Ctrl Pts',(-183.717166718273,96.0331520763448,2.99925051740835));
#27592=CARTESIAN_POINT('Ctrl Pts',(-183.674920024759,96.0732153826263,2.90364281121743));
#27593=CARTESIAN_POINT('Ctrl Pts',(-183.647332236574,96.0993773829103,2.84120940098035));
#27594=CARTESIAN_POINT('Ctrl Pts',(-183.620385155488,96.1249086081634,2.77812375522392));
#27595=CARTESIAN_POINT('Ctrl Pts',(-183.594152714823,96.1497420997336,2.71444332769558));
#27596=CARTESIAN_POINT('Ctrl Pts',(-183.552513710988,96.1891605382974,2.61336277632992));
#27597=CARTESIAN_POINT('Ctrl Pts',(-183.512667688487,96.2268302669331,2.5107665238383));
#27598=CARTESIAN_POINT('Ctrl Pts',(-183.474859837213,96.262532942592,2.40684095748967));
#27599=CARTESIAN_POINT('Ctrl Pts',(-183.446737682174,96.2890892304089,2.32953926509386));
#27600=CARTESIAN_POINT('Ctrl Pts',(-183.419742343131,96.3145579714235,2.25150195220109));
#27601=CARTESIAN_POINT('Ctrl Pts',(-183.393961050788,96.3388617174235,2.17280303683206));
#27602=CARTESIAN_POINT('Ctrl Pts',(-183.359580666358,96.3712717347123,2.06785488572363));
#27603=CARTESIAN_POINT('Ctrl Pts',(-183.327343569224,96.4016267776895,1.96172200413313));
#27604=CARTESIAN_POINT('Ctrl Pts',(-183.297389795937,96.4298084395749,1.8542397954829));
#27605=CARTESIAN_POINT('Ctrl Pts',(-183.274245858352,96.4515831461358,1.77119311202647));
#27606=CARTESIAN_POINT('Ctrl Pts',(-183.252464429557,96.4720609088697,1.68734163313003));
#27607=CARTESIAN_POINT('Ctrl Pts',(-183.232098245116,96.4911976665063,1.60262357057942));
#27608=CARTESIAN_POINT('Ctrl Pts',(-183.216389907906,96.5059577529103,1.53728094843953));
#27609=CARTESIAN_POINT('Ctrl Pts',(-183.201534766402,96.5199094694207,1.47135146558728));
#27610=CARTESIAN_POINT('Ctrl Pts',(-183.187602228551,96.5329901074898,1.40511236999388));
#27611=CARTESIAN_POINT('Ctrl Pts',(-183.168469031447,96.5509534124586,1.31414791789888));
#27612=CARTESIAN_POINT('Ctrl Pts',(-183.151038568884,96.5673071210697,1.22241879048284));
#27613=CARTESIAN_POINT('Ctrl Pts',(-183.135478803873,96.5818992004815,1.13048589166228));
#27614=CARTESIAN_POINT('Ctrl Pts',(-183.127438973994,96.5894390210347,1.08298357616052));
#27615=CARTESIAN_POINT('Ctrl Pts',(-183.119898495986,96.5965085951852,1.03542593039518));
#27616=CARTESIAN_POINT('Ctrl Pts',(-183.112880159761,96.6030872601668,0.987885042250572));
#27617=CARTESIAN_POINT('Ctrl Pts',(-183.094272288311,96.6205294214393,0.861838824608398));
#27618=CARTESIAN_POINT('Ctrl Pts',(-183.079158190004,96.6346871142076,0.735294438806359));
#27619=CARTESIAN_POINT('Ctrl Pts',(-183.067609370826,96.6455017519546,0.607979113572891));
#27620=CARTESIAN_POINT('Ctrl Pts',(-183.059751403966,96.6528601722144,0.521352109460987));
#27621=CARTESIAN_POINT('Ctrl Pts',(-183.053544641283,96.6586702885726,0.434367916619133));
#27622=CARTESIAN_POINT('Ctrl Pts',(-183.049021241499,96.6629044452172,0.346936379531023));
#27623=CARTESIAN_POINT('Ctrl Pts',(-183.043938087641,96.6676625631615,0.24868551154289));
#27624=CARTESIAN_POINT('Ctrl Pts',(-183.041042521995,96.6703728479844,0.149377453584831));
#27625=CARTESIAN_POINT('Ctrl Pts',(-183.040310525973,96.6710579738602,0.0500714675686074));
#27626=CARTESIAN_POINT('Ctrl Pts',(-183.040187486682,96.6711731348712,0.0333793849144663));
#27627=CARTESIAN_POINT('Ctrl Pts',(-183.040125617894,96.6712310386364,0.0166872567960485));
#27628=CARTESIAN_POINT('Ctrl Pts',(-183.040124856982,96.67123174467,-7.3835382252696E-10));
#27629=CARTESIAN_POINT('',(6.58230156589418E-15,207.,-1.83697019872103E-15));
#27630=CARTESIAN_POINT('Origin',(0.,0.,-1.83697019872103E-15));
#27631=CARTESIAN_POINT('',(0.,222.,-15.));
#27632=CARTESIAN_POINT('Origin',(0.,222.,0.));
#27633=CARTESIAN_POINT('Origin',(0.,222.,0.));
#27634=CARTESIAN_POINT('',(-188.497895047951,-91.2584808544846,-8.18007173203753));
#27635=CARTESIAN_POINT('Ctrl Pts',(-183.040047979333,96.6713030620956,-1.78040965343625E-11));
#27636=CARTESIAN_POINT('Ctrl Pts',(-183.040047979334,96.671303062095,-0.290717296796128));
#27637=CARTESIAN_POINT('Ctrl Pts',(-183.058923419162,96.6536479752409,-0.578335867620054));
#27638=CARTESIAN_POINT('Ctrl Pts',(-183.132297130496,96.5849017443526,-1.14764968196531));
#27639=CARTESIAN_POINT('Ctrl Pts',(-183.187136433235,96.5334867370368,-1.42960539277542));
#27640=CARTESIAN_POINT('Ctrl Pts',(-183.395676877553,96.3374453080213,-2.24595901383476));
#27641=CARTESIAN_POINT('Ctrl Pts',(-183.596179288576,96.148378129504,-2.76253014436806));
#27642=CARTESIAN_POINT('Ctrl Pts',(-183.948385873179,95.813304980467,-3.47403718087876));
#27643=CARTESIAN_POINT('Ctrl Pts',(-184.074723247574,95.6927020889136,-3.70196303508026));
#27644=CARTESIAN_POINT('Ctrl Pts',(-184.342135655567,95.4362859797969,-4.14231049014845));
#27645=CARTESIAN_POINT('Ctrl Pts',(-184.483878266456,95.2998256542781,-4.35559560516305));
#27646=CARTESIAN_POINT('Ctrl Pts',(-184.922137729314,94.8758603284929,-4.96776945688272));
#27647=CARTESIAN_POINT('Ctrl Pts',(-185.231024285832,94.5744209337779,-5.3396847793381));
#27648=CARTESIAN_POINT('Ctrl Pts',(-186.189742337321,93.6287929397982,-6.38062863151832));
#27649=CARTESIAN_POINT('Ctrl Pts',(-186.870931608401,92.9438803352724,-6.97616626868284));
#27650=CARTESIAN_POINT('Ctrl Pts',(-187.922915121028,91.8603562891812,-7.7814123143153));
#27651=CARTESIAN_POINT('Ctrl Pts',(-188.27976116909,91.4886432157324,-8.03501547234262));
#27652=CARTESIAN_POINT('Ctrl Pts',(-188.991709907376,90.7381517492508,-8.51093004128364));
#27653=CARTESIAN_POINT('Ctrl Pts',(-189.347946938551,90.3582289492531,-8.73415029064059));
#27654=CARTESIAN_POINT('Ctrl Pts',(-190.415704618364,89.2057861435712,-9.36797876968955));
#27655=CARTESIAN_POINT('Ctrl Pts',(-191.126187452397,88.4206612756743,-9.74317222706952));
#27656=CARTESIAN_POINT('Ctrl Pts',(-192.538651519066,86.8210527672942,-10.4260665657394));
#27657=CARTESIAN_POINT('Ctrl Pts',(-193.240691367808,86.0065197832478,-10.7334743463981));
#27658=CARTESIAN_POINT('Ctrl Pts',(-195.328969811832,83.522361710867,-11.5774799750461));
#27659=CARTESIAN_POINT('Ctrl Pts',(-196.697140045752,81.8123666295429,-12.0369899115148));
#27660=CARTESIAN_POINT('Ctrl Pts',(-198.701009621295,79.1739133145013,-12.6241943015858));
#27661=CARTESIAN_POINT('Ctrl Pts',(-199.360982676768,78.2821187303764,-12.8025189004934));
#27662=CARTESIAN_POINT('Ctrl Pts',(-200.663565069239,76.4745743432818,-13.1297934395841));
#27663=CARTESIAN_POINT('Ctrl Pts',(-201.307303606054,75.5571516619106,-13.2789601805961));
#27664=CARTESIAN_POINT('Ctrl Pts',(-203.201516047313,72.7832478647282,-13.6867621695905));
#27665=CARTESIAN_POINT('Ctrl Pts',(-204.413700546118,70.9075282912295,-13.9060360996326));
#27666=CARTESIAN_POINT('Ctrl Pts',(-207.899657365585,65.2035836701327,-14.4507645550931));
#27667=CARTESIAN_POINT('Ctrl Pts',(-210.023128099383,61.2987994893877,-14.6650896802637));
#27668=CARTESIAN_POINT('Ctrl Pts',(-213.870276136955,53.2915163853001,-14.933497953333));
#27669=CARTESIAN_POINT('Ctrl Pts',(-215.594021132889,49.1889740960755,-14.985853687648));
#27670=CARTESIAN_POINT('Ctrl Pts',(-217.873399431556,42.8864129541246,-15.0033037809541));
#27671=CARTESIAN_POINT('Ctrl Pts',(-218.582069674932,40.7607166635472,-14.9986689688532));
#27672=CARTESIAN_POINT('Ctrl Pts',(-219.56675968207,37.5343872263211,-14.9819099628708));
#27673=CARTESIAN_POINT('Ctrl Pts',(-219.8822170261,36.4514838658265,-14.9746676310821));
#27674=CARTESIAN_POINT('Ctrl Pts',(-220.483358450152,34.2853764016843,-14.9578746973126));
#27675=CARTESIAN_POINT('Ctrl Pts',(-220.769465484776,33.2008912844799,-14.9483204745317));
#27676=CARTESIAN_POINT('Ctrl Pts',(-222.12855866699,27.7713853384315,-14.8968645760071));
#27677=CARTESIAN_POINT('Ctrl Pts',(-222.987787020107,23.4051756849622,-14.8447490296456));
#27678=CARTESIAN_POINT('Ctrl Pts',(-224.263142252711,14.6286399575493,-14.7581200953001));
#27679=CARTESIAN_POINT('Ctrl Pts',(-224.67923658837,10.2183109541443,-14.7235458426584));
#27680=CARTESIAN_POINT('Ctrl Pts',(-225.067487120359,1.35335614042816,-14.6914557569397));
#27681=CARTESIAN_POINT('Ctrl Pts',(-225.039680369902,-3.10126619891411,
-14.6939820956571));
#27682=CARTESIAN_POINT('Ctrl Pts',(-224.65412178184,-9.81750421703877,-14.7254343338351));
#27683=CARTESIAN_POINT('Ctrl Pts',(-224.4672482405,-12.0685257533435,-14.740436703992));
#27684=CARTESIAN_POINT('Ctrl Pts',(-223.981935807087,-16.5303006920475,
-14.7768220386414));
#27685=CARTESIAN_POINT('Ctrl Pts',(-223.683613303296,-18.7451256741302,
-14.7981937237368));
#27686=CARTESIAN_POINT('Ctrl Pts',(-222.625392381006,-25.3424864211294,
-14.8664210701889));
#27687=CARTESIAN_POINT('Ctrl Pts',(-221.702647102239,-29.6780260824246,
-14.9179126495301));
#27688=CARTESIAN_POINT('Ctrl Pts',(-219.432103438233,-38.226379286061,-14.9914332557902));
#27689=CARTESIAN_POINT('Ctrl Pts',(-218.084289955228,-42.4391887915816,
-15.0136856420233));
#27690=CARTESIAN_POINT('Ctrl Pts',(-214.960123702443,-50.7409884267741,
-14.9681429282199));
#27691=CARTESIAN_POINT('Ctrl Pts',(-213.183822160821,-54.8299944921915,
-14.9011481177155));
#27692=CARTESIAN_POINT('Ctrl Pts',(-210.685097784923,-59.8607475849498,
-14.702829183641));
#27693=CARTESIAN_POINT('Ctrl Pts',(-210.170653953151,-60.8642286915694,
-14.6572311370428));
#27694=CARTESIAN_POINT('Ctrl Pts',(-209.118711926601,-62.8532204215151,
-14.5527940286245));
#27695=CARTESIAN_POINT('Ctrl Pts',(-208.580972841412,-63.8393132496125,
-14.4939525317814));
#27696=CARTESIAN_POINT('Ctrl Pts',(-206.932956196544,-66.7723267156479,
-14.2945370605171));
#27697=CARTESIAN_POINT('Ctrl Pts',(-205.78787826466,-68.6940106709314,-14.1313021234452));
#27698=CARTESIAN_POINT('Ctrl Pts',(-203.40751840668,-72.4691497536957,-13.7237471362256));
#27699=CARTESIAN_POINT('Ctrl Pts',(-202.172215713411,-74.3226190289864,
-13.4796454873293));
#27700=CARTESIAN_POINT('Ctrl Pts',(-199.614242706283,-77.9593665780488,
-12.880290719481));
#27701=CARTESIAN_POINT('Ctrl Pts',(-198.291521481218,-79.7426835304235,
-12.5256047378343));
#27702=CARTESIAN_POINT('Ctrl Pts',(-196.24496263622,-82.3622188310058,-11.872433441665));
#27703=CARTESIAN_POINT('Ctrl Pts',(-195.553967137143,-83.2240348135499,
-11.6347489559485));
#27704=CARTESIAN_POINT('Ctrl Pts',(-194.162346915831,-84.9164771058137,
-11.1125529770436));
#27705=CARTESIAN_POINT('Ctrl Pts',(-193.460866402951,-85.7481952744176,
-10.8278555945698));
#27706=CARTESIAN_POINT('Ctrl Pts',(-192.050013622452,-87.3804628822538,
-10.1985906850403));
#27707=CARTESIAN_POINT('Ctrl Pts',(-191.340598963084,-88.1810474344335,
-9.85419988852607));
#27708=CARTESIAN_POINT('Ctrl Pts',(-189.919091050928,-89.7474499656185,
-9.08558654970619));
#27709=CARTESIAN_POINT('Ctrl Pts',(-189.206880667753,-90.5133679110211,
-8.66185957465181));
#27710=CARTESIAN_POINT('Ctrl Pts',(-188.497895047951,-91.2584808544846,
-8.18007173203753));
#27711=CARTESIAN_POINT('Ctrl Pts',(-188.497895047951,-91.2584808544846,
-8.18007173203754));
#27712=CARTESIAN_POINT('Ctrl Pts',(-188.300062055738,-91.4663946950838,
-8.0456352528558));
#27713=CARTESIAN_POINT('Ctrl Pts',(-188.103136583577,-91.6719902155658,
-7.90706781866979));
#27714=CARTESIAN_POINT('Ctrl Pts',(-187.907384188659,-91.8750715954411,
-7.76381635884333));
#27715=CARTESIAN_POINT('Ctrl Pts',(-187.718661179823,-92.0708604084685,
-7.6257089986259));
#27716=CARTESIAN_POINT('Ctrl Pts',(-187.531028538814,-92.2643124052881,
-7.48324791185683));
#27717=CARTESIAN_POINT('Ctrl Pts',(-187.344714547772,-92.455262437099,-7.33598118338943));
#27718=CARTESIAN_POINT('Ctrl Pts',(-187.176146527014,-92.6280249266267,
-7.20274126510646));
#27719=CARTESIAN_POINT('Ctrl Pts',(-187.008650204035,-92.7987460149388,
-7.0656087741307));
#27720=CARTESIAN_POINT('Ctrl Pts',(-186.842467463592,-92.9672410175639,
-6.92394517460035));
#27721=CARTESIAN_POINT('Ctrl Pts',(-186.799612610027,-93.0106921524095,
-6.88741326522613));
#27722=CARTESIAN_POINT('Ctrl Pts',(-186.75684505207,-93.0539953071172,-6.85058028783488));
#27723=CARTESIAN_POINT('Ctrl Pts',(-186.714168812212,-93.0971474350744,
-6.81343583506232));
#27724=CARTESIAN_POINT('Ctrl Pts',(-186.568967960517,-93.2439674396628,
-6.68705623376176));
#27725=CARTESIAN_POINT('Ctrl Pts',(-186.424842134083,-93.3890455019234,
-6.55710606451584));
#27726=CARTESIAN_POINT('Ctrl Pts',(-186.281951647043,-93.5322032134759,
-6.42315381606293));
#27727=CARTESIAN_POINT('Ctrl Pts',(-186.257009039101,-93.5571924674637,
-6.3997714448129));
#27728=CARTESIAN_POINT('Ctrl Pts',(-186.231992582235,-93.582233475522,-6.3761612335205));
#27729=CARTESIAN_POINT('Ctrl Pts',(-186.206930421579,-93.6072983045629,
-6.35234366750294));
#27730=CARTESIAN_POINT('Ctrl Pts',(-186.144618582895,-93.6696167776295,
-6.29312625397292));
#27731=CARTESIAN_POINT('Ctrl Pts',(-186.082020331053,-93.73208556107,-6.23264317803972));
#27732=CARTESIAN_POINT('Ctrl Pts',(-186.019574250509,-93.7942745571904,
-6.17119264600906));
#27733=CARTESIAN_POINT('Ctrl Pts',(-185.963251794942,-93.8503651387019,
-6.1157681128792));
#27734=CARTESIAN_POINT('Ctrl Pts',(-185.907053155763,-93.9062281788253,
-6.05955663501713));
#27735=CARTESIAN_POINT('Ctrl Pts',(-185.851294277388,-93.961557772832,-6.00281180135348));
#27736=CARTESIAN_POINT('Ctrl Pts',(-185.749818148972,-94.0622526424254,
-5.8995413232585));
#27737=CARTESIAN_POINT('Ctrl Pts',(-185.64944798569,-94.1615675588845,-5.79419527240436));
#27738=CARTESIAN_POINT('Ctrl Pts',(-185.550310946567,-94.2593715002356,
-5.68653596243487));
#27739=CARTESIAN_POINT('Ctrl Pts',(-185.453240346919,-94.3551367895654,
-5.58112073247738));
#27740=CARTESIAN_POINT('Ctrl Pts',(-185.357352047033,-94.4494534467525,
-5.473487596431));
#27741=CARTESIAN_POINT('Ctrl Pts',(-185.262760907272,-94.5422101471869,
-5.36346162345762));
#27742=CARTESIAN_POINT('Ctrl Pts',(-185.207680102582,-94.5962227504107,
-5.29939305272703));
#27743=CARTESIAN_POINT('Ctrl Pts',(-185.153039048079,-94.649706625106,-5.23451403425678));
#27744=CARTESIAN_POINT('Ctrl Pts',(-185.098859601402,-94.7026416531689,
-5.16879796046587));
#27745=CARTESIAN_POINT('Ctrl Pts',(-185.074330592064,-94.7266072688649,
-5.13904589973869));
#27746=CARTESIAN_POINT('Ctrl Pts',(-185.049896921581,-94.7504597611539,
-5.10911917048002));
#27747=CARTESIAN_POINT('Ctrl Pts',(-185.025562001606,-94.7741960738258,
-5.07900945369665));
#27748=CARTESIAN_POINT('Ctrl Pts',(-184.946413429458,-94.8513976942973,
-4.98107853410751));
#27749=CARTESIAN_POINT('Ctrl Pts',(-184.868310362198,-94.9273894652854,
-4.88123324740708));
#27750=CARTESIAN_POINT('Ctrl Pts',(-184.791382991276,-95.002060866969,-4.77925814868048));
#27751=CARTESIAN_POINT('Ctrl Pts',(-184.714455620355,-95.0767322686525,
-4.67728304995388));
#27752=CARTESIAN_POINT('Ctrl Pts',(-184.638704007293,-95.1500832519385,
-4.57317788266935));
#27753=CARTESIAN_POINT('Ctrl Pts',(-184.564246641858,-95.2220151025974,
-4.46678202474539));
#27754=CARTESIAN_POINT('Ctrl Pts',(-184.497056056092,-95.2869266550372,
-4.37077003217547));
#27755=CARTESIAN_POINT('Ctrl Pts',(-184.430943906992,-95.3506568984757,
-4.2729026001225));
#27756=CARTESIAN_POINT('Ctrl Pts',(-184.366226272981,-95.412919659581,-4.17327681029906));
#27757=CARTESIAN_POINT('Ctrl Pts',(-184.334563669764,-95.4433812351646,
-4.12453566112887));
#27758=CARTESIAN_POINT('Ctrl Pts',(-184.303234341527,-95.4734920445134,
-4.07537395381293));
#27759=CARTESIAN_POINT('Ctrl Pts',(-184.272272264877,-95.5032214550723,
-4.0258048980475));
#27760=CARTESIAN_POINT('Ctrl Pts',(-184.206611201955,-95.5662684114961,
-3.92068414253747));
#27761=CARTESIAN_POINT('Ctrl Pts',(-184.142567466176,-95.6276314764618,
-3.81366921333017));
#27762=CARTESIAN_POINT('Ctrl Pts',(-184.080412946787,-95.6870699231794,
-3.70484958990335));
#27763=CARTESIAN_POINT('Ctrl Pts',(-184.072028903129,-95.6950875948971,
-3.69017087494246));
#27764=CARTESIAN_POINT('Ctrl Pts',(-184.063679179314,-95.7030702979177,
-3.67545934343523));
#27765=CARTESIAN_POINT('Ctrl Pts',(-184.055364391027,-95.71101748865,-3.66071523418955));
#27766=CARTESIAN_POINT('Ctrl Pts',(-183.999462471019,-95.7644479796339,
-3.56158775346746));
#27767=CARTESIAN_POINT('Ctrl Pts',(-183.944910782877,-95.8164915916668,
-3.46059627411805));
#27768=CARTESIAN_POINT('Ctrl Pts',(-183.892007949902,-95.8668829533374,
-3.35779889575907));
#27769=CARTESIAN_POINT('Ctrl Pts',(-183.83899400497,-95.9173801521151,-3.25478561180084));
#27770=CARTESIAN_POINT('Ctrl Pts',(-183.787635848404,-95.9662181505276,
-3.14995885084012));
#27771=CARTESIAN_POINT('Ctrl Pts',(-183.738196574503,-96.0131639139981,
-3.04339088491695));
#27772=CARTESIAN_POINT('Ctrl Pts',(-183.70441834109,-96.0452385144339,-2.97058080209866));
#27773=CARTESIAN_POINT('Ctrl Pts',(-183.671535061622,-96.0764305291934,
-2.8969582139391));
#27774=CARTESIAN_POINT('Ctrl Pts',(-183.639620656277,-96.106674727365,-2.82254979915783));
#27775=CARTESIAN_POINT('Ctrl Pts',(-183.625882932619,-96.1196935015595,
-2.79052030560972));
#27776=CARTESIAN_POINT('Ctrl Pts',(-183.612325271825,-96.1325356385398,
-2.75834550238426));
#27777=CARTESIAN_POINT('Ctrl Pts',(-183.598953725412,-96.1451958361621,
-2.72602941545094));
#27778=CARTESIAN_POINT('Ctrl Pts',(-183.559671567108,-96.1823882349924,
-2.63109307798464));
#27779=CARTESIAN_POINT('Ctrl Pts',(-183.522065131717,-96.2179455935306,
-2.5352045733376));
#27780=CARTESIAN_POINT('Ctrl Pts',(-183.486282382413,-96.2517422824135,
-2.43826741633881));
#27781=CARTESIAN_POINT('Ctrl Pts',(-183.4507080064,-96.2853421634085,-2.34189475242377));
#27782=CARTESIAN_POINT('Ctrl Pts',(-183.416936172958,-96.3172017871073,
-2.24448556910026));
#27783=CARTESIAN_POINT('Ctrl Pts',(-183.385084418382,-96.3472227051745,
-2.14598002821041));
#27784=CARTESIAN_POINT('Ctrl Pts',(-183.353419282572,-96.3770677313077,
-2.04805162923407));
#27785=CARTESIAN_POINT('Ctrl Pts',(-183.323651806033,-96.4050955186365,
-1.94903966326626));
#27786=CARTESIAN_POINT('Ctrl Pts',(-183.295869501762,-96.4312344867279,
-1.84892047240775));
#27787=CARTESIAN_POINT('Ctrl Pts',(-183.276527910854,-96.4494320135649,
-1.77921911096964));
#27788=CARTESIAN_POINT('Ctrl Pts',(-183.258147894583,-96.4667146064943,
-1.70898184056822));
#27789=CARTESIAN_POINT('Ctrl Pts',(-183.240750872462,-96.4830654179867,
-1.6382108706281));
#27790=CARTESIAN_POINT('Ctrl Pts',(-183.227158803033,-96.4958400965205,
-1.58291842285402));
#27791=CARTESIAN_POINT('Ctrl Pts',(-183.214149487226,-96.5080622644032,
-1.52710078869208));
#27792=CARTESIAN_POINT('Ctrl Pts',(-183.201778674498,-96.5196811723908,
-1.47094697429921));
#27793=CARTESIAN_POINT('Ctrl Pts',(-183.182833430955,-96.537474913706,-1.38495038595907));
#27794=CARTESIAN_POINT('Ctrl Pts',(-183.165335520778,-96.5538973659424,
-1.29792703960836));
#27795=CARTESIAN_POINT('Ctrl Pts',(-183.149458653825,-96.5687909504186,
-1.21032489975144));
#27796=CARTESIAN_POINT('Ctrl Pts',(-183.138155472576,-96.5793941056436,
-1.1479585104899));
#27797=CARTESIAN_POINT('Ctrl Pts',(-183.12767372067,-96.5892225243258,-1.08529737450488));
#27798=CARTESIAN_POINT('Ctrl Pts',(-183.118075583124,-96.5982196502656,
-1.02248733130099));
#27799=CARTESIAN_POINT('Ctrl Pts',(-183.103912230031,-96.6114961292588,
-0.929802597894992));
#27800=CARTESIAN_POINT('Ctrl Pts',(-183.091641950435,-96.6229920891114,
-0.836874057660911));
#27801=CARTESIAN_POINT('Ctrl Pts',(-183.081282937533,-96.6326945944338,
-0.743544356439005));
#27802=CARTESIAN_POINT('Ctrl Pts',(-183.069236032265,-96.6439780211072,
-0.635007560508499));
#27803=CARTESIAN_POINT('Ctrl Pts',(-183.059794785879,-96.6528172613218,
-0.526131955687998));
#27804=CARTESIAN_POINT('Ctrl Pts',(-183.05299282205,-96.6591851125678,-0.416662911030544));
#27805=CARTESIAN_POINT('Ctrl Pts',(-183.052127587993,-96.6599951259555,
-0.402738058159433));
#27806=CARTESIAN_POINT('Ctrl Pts',(-183.051305108022,-96.660765104651,-0.388803583785994));
#27807=CARTESIAN_POINT('Ctrl Pts',(-183.050525494592,-96.6614949518932,
-0.374858946693551));
#27808=CARTESIAN_POINT('Ctrl Pts',(-183.045113804408,-96.6665611898578,
-0.278062184637631));
#27809=CARTESIAN_POINT('Ctrl Pts',(-183.041826513527,-96.669638755822,-0.180534200127789));
#27810=CARTESIAN_POINT('Ctrl Pts',(-183.040628942412,-96.6707598747363,
-0.0830679383035017));
#27811=CARTESIAN_POINT('Ctrl Pts',(-183.040288591815,-96.6710784975613,
-0.0553679545761854));
#27812=CARTESIAN_POINT('Ctrl Pts',(-183.040117202872,-96.6712389343265,
-0.0276727228799533));
#27813=CARTESIAN_POINT('Ctrl Pts',(-183.04011439547,-96.6712415351879,1.37667022226395E-9));
#27814=CARTESIAN_POINT('Ctrl Pts',(-188.957144201311,90.8303388274957,5.37500533271896));
#27815=CARTESIAN_POINT('Ctrl Pts',(-188.724920768398,91.1301703614817,6.55330325436076));
#27816=CARTESIAN_POINT('Ctrl Pts',(-189.086176933001,91.8055258010517,7.52572239671998));
#27817=CARTESIAN_POINT('Ctrl Pts',(-188.593855532332,91.2997460800671,5.17875473137162));
#27818=CARTESIAN_POINT('Ctrl Pts',(-188.358392135328,91.6013100563716,6.30706395511774));
#27819=CARTESIAN_POINT('Ctrl Pts',(-188.672178961879,92.2572808761228,7.25093082992469));
#27820=CARTESIAN_POINT('Ctrl Pts',(-188.230166171018,91.7638380268742,4.96746400526744));
#27821=CARTESIAN_POINT('Ctrl Pts',(-187.990226260873,92.0686730594487,6.04280873676479));
#27822=CARTESIAN_POINT('Ctrl Pts',(-188.25791121472,92.7031848330253,6.95510627280203));
#27823=CARTESIAN_POINT('Ctrl Pts',(-187.539693143008,92.6343805277346,4.52454205690639));
#27824=CARTESIAN_POINT('Ctrl Pts',(-187.291011725483,92.9455045001231,5.49198587002716));
#27825=CARTESIAN_POINT('Ctrl Pts',(-187.471668401951,93.5383530782691,6.3349561219722));
#27826=CARTESIAN_POINT('Ctrl Pts',(-187.212048839638,93.0429197330079,4.29662107665932));
#27827=CARTESIAN_POINT('Ctrl Pts',(-186.959279127768,93.3569115666992,5.21014878574447));
#27828=CARTESIAN_POINT('Ctrl Pts',(-187.098702415434,93.9297277637807,6.01583633368207));
#27829=CARTESIAN_POINT('Ctrl Pts',(-186.564202659971,93.8422554296375,3.7905424310452));
#27830=CARTESIAN_POINT('Ctrl Pts',(-186.303378595483,94.1617059643359,4.58745384323657));
#27831=CARTESIAN_POINT('Ctrl Pts',(-186.361481988203,94.6944082162028,5.30725885908418));
#27832=CARTESIAN_POINT('Ctrl Pts',(-186.246046490499,94.2305182540288,3.51471556151069));
#27833=CARTESIAN_POINT('Ctrl Pts',(-185.981150185696,94.552750507534,4.24970897101787));
#27834=CARTESIAN_POINT('Ctrl Pts',(-185.999555835803,95.0652888521504,4.92106466935472));
#27835=CARTESIAN_POINT('Ctrl Pts',(-185.7860440826,94.7865211755072,3.04374365253442));
#27836=CARTESIAN_POINT('Ctrl Pts',(-185.51477702092,95.1132429797568,3.67482442913072));
#27837=CARTESIAN_POINT('Ctrl Pts',(-185.476427677548,95.5956987820616,4.26164147337986));
#27838=CARTESIAN_POINT('Ctrl Pts',(-185.635237128339,94.9678695342472,2.87648994589474));
#27839=CARTESIAN_POINT('Ctrl Pts',(-185.362056916117,95.2958407269429,3.47137285105012));
#27840=CARTESIAN_POINT('Ctrl Pts',(-185.304953205109,95.7685766079577,4.02746418701679));
#27841=CARTESIAN_POINT('Ctrl Pts',(-185.346408587176,95.3136337587549,2.51967239257564));
#27842=CARTESIAN_POINT('Ctrl Pts',(-185.069604964524,95.643921849378,3.03821885310616));
#27843=CARTESIAN_POINT('Ctrl Pts',(-184.97658882459,96.0979829082245,3.52787252597041));
#27844=CARTESIAN_POINT('Ctrl Pts',(-185.20795883318,95.4785673522034,2.32993303963118));
#27845=CARTESIAN_POINT('Ctrl Pts',(-184.929379865569,95.8100014195192,2.80832193017784));
#27846=CARTESIAN_POINT('Ctrl Pts',(-184.819211984195,96.2550053176917,3.26221242414813));
#27847=CARTESIAN_POINT('Ctrl Pts',(-184.949109662307,95.7857342654447,1.91734928765954));
#27848=CARTESIAN_POINT('Ctrl Pts',(-184.667275037263,96.1192146731736,2.30933190506252));
#27849=CARTESIAN_POINT('Ctrl Pts',(-184.525013064704,96.5472768103603,2.68454085282217));
#27850=CARTESIAN_POINT('Ctrl Pts',(-184.827448410629,95.9294455889528,1.69197258199757));
#27851=CARTESIAN_POINT('Ctrl Pts',(-184.544028383669,96.2639439959695,2.03717831284139));
#27852=CARTESIAN_POINT('Ctrl Pts',(-184.3867574195,96.6839296134637,2.36898381675622));
#27853=CARTESIAN_POINT('Ctrl Pts',(-184.673157550248,96.1111707509329,1.32666686830212));
#27854=CARTESIAN_POINT('Ctrl Pts',(-184.387725058793,96.4469529143824,1.59654749755515));
#27855=CARTESIAN_POINT('Ctrl Pts',(-184.21143808209,96.8566566608848,1.85750776184721));
#27856=CARTESIAN_POINT('Ctrl Pts',(-184.626384664622,96.1661612824647,1.20034830913053));
#27857=CARTESIAN_POINT('Ctrl Pts',(-184.340354066678,96.5023171881443,1.44433813660881));
#27858=CARTESIAN_POINT('Ctrl Pts',(-184.158293562368,96.9089107493774,1.68064518391667));
#27859=CARTESIAN_POINT('Ctrl Pts',(-184.544557060113,96.2622563647223,0.936341947650762));
#27860=CARTESIAN_POINT('Ctrl Pts',(-184.257494308414,96.5990477794699,1.12641432764746));
#27861=CARTESIAN_POINT('Ctrl Pts',(-184.065322417016,97.0002089202945,1.31100161190584));
#27862=CARTESIAN_POINT('Ctrl Pts',(-184.509590436998,96.3032573605489,0.798204058161918));
#27863=CARTESIAN_POINT('Ctrl Pts',(-184.222078190747,96.6403292797306,0.960133989517193));
#27864=CARTESIAN_POINT('Ctrl Pts',(-184.025595889726,97.0391546118712,1.11759042863826));
#27865=CARTESIAN_POINT('Ctrl Pts',(-184.456423260012,96.3655603217114,0.518880062316245));
#27866=CARTESIAN_POINT('Ctrl Pts',(-184.168239976604,96.7030436386975,0.624058853398732));
#27867=CARTESIAN_POINT('Ctrl Pts',(-183.96519246775,97.0983289670991,0.726500176433084));
#27868=CARTESIAN_POINT('Ctrl Pts',(-184.43780991789,96.3873480254583,0.376560788584548));
#27869=CARTESIAN_POINT('Ctrl Pts',(-184.149386424996,96.7249811721857,0.45285850256557));
#27870=CARTESIAN_POINT('Ctrl Pts',(-183.944046539593,97.1190192634854,0.527234512604526));
#27871=CARTESIAN_POINT('Ctrl Pts',(-184.418424799205,96.4100379276536,0.0859862665940266));
#27872=CARTESIAN_POINT('Ctrl Pts',(-184.129756564253,96.7478207757289,0.103410177548531));
#27873=CARTESIAN_POINT('Ctrl Pts',(-183.922023861298,97.1405661466642,0.120392057990099));
#27874=CARTESIAN_POINT('Ctrl Pts',(-184.417917263625,96.4106316699318,-0.0638962092285304));
#27875=CARTESIAN_POINT('Ctrl Pts',(-184.129242485696,96.7484185900842,-0.0768454065926074));
#27876=CARTESIAN_POINT('Ctrl Pts',(-183.921447280066,97.1411299348213,-0.0894630792312966));
#27877=CARTESIAN_POINT('Ctrl Pts',(-184.435598572149,96.3899366351428,-0.355921346913274));
#27878=CARTESIAN_POINT('Ctrl Pts',(-184.147147026983,96.7275870182977,-0.428034207439262));
#27879=CARTESIAN_POINT('Ctrl Pts',(-183.941534307246,97.1214775080755,-0.498336585883369));
#27880=CARTESIAN_POINT('Ctrl Pts',(-184.453495989889,96.3689882627064,-0.499360335068101));
#27881=CARTESIAN_POINT('Ctrl Pts',(-184.165275543997,96.7064944488072,-0.600578183941243));
#27882=CARTESIAN_POINT('Ctrl Pts',(-183.961866858988,97.1015844491156,-0.699169996799552));
#27883=CARTESIAN_POINT('Ctrl Pts',(-184.505728755164,96.3077846419852,-0.781557979895856));
#27884=CARTESIAN_POINT('Ctrl Pts',(-184.218167565914,96.6448867100655,-0.94010099938254));
#27885=CARTESIAN_POINT('Ctrl Pts',(-184.021208554627,97.0434548337247,-1.09428373408145));
#27886=CARTESIAN_POINT('Ctrl Pts',(-184.540234799446,96.2673269623919,-0.920237385586888));
#27887=CARTESIAN_POINT('Ctrl Pts',(-184.253117035716,96.6041524436365,-1.10702701224397));
#27888=CARTESIAN_POINT('Ctrl Pts',(-184.06041170346,97.0050256725195,-1.28845311054166));
#27889=CARTESIAN_POINT('Ctrl Pts',(-184.620686872807,96.1728572150355,-1.18387310682941));
#27890=CARTESIAN_POINT('Ctrl Pts',(-184.334583941818,96.5090579829018,-1.42449083732315));
#27891=CARTESIAN_POINT('Ctrl Pts',(-184.151819680695,96.9152730760786,-1.65757773666664));
#27892=CARTESIAN_POINT('Ctrl Pts',(-184.666866291424,96.1185715284399,-1.31029463806153));
#27893=CARTESIAN_POINT('Ctrl Pts',(-184.381354073376,96.454403175623,-1.5768166801151));
#27894=CARTESIAN_POINT('Ctrl Pts',(-184.204289665826,96.863689736492,-1.83458448860681));
#27895=CARTESIAN_POINT('Ctrl Pts',(-184.768797731556,95.9985328752646,-1.55440284628578));
#27896=CARTESIAN_POINT('Ctrl Pts',(-184.484570250941,96.3335691070844,-1.87111429108252));
#27897=CARTESIAN_POINT('Ctrl Pts',(-184.320112912034,96.7495971531963,-2.17636805559542));
#27898=CARTESIAN_POINT('Ctrl Pts',(-184.824880454895,95.932388707861,-1.67265647736271));
#27899=CARTESIAN_POINT('Ctrl Pts',(-184.541367291036,96.2669769912313,-2.0137851155555));
#27900=CARTESIAN_POINT('Ctrl Pts',(-184.383841997721,96.6867158385967,-2.34193868595053));
#27901=CARTESIAN_POINT('Ctrl Pts',(-185.002343333799,95.7226659996551,-2.01149464431596));
#27902=CARTESIAN_POINT('Ctrl Pts',(-184.721154715952,96.0557554309112,-2.42308663113885));
#27903=CARTESIAN_POINT('Ctrl Pts',(-184.585513418963,96.4872808224781,-2.81635673893943));
#27904=CARTESIAN_POINT('Ctrl Pts',(-185.132392337656,95.5684417093648,-2.21657750656061));
#27905=CARTESIAN_POINT('Ctrl Pts',(-184.852882048359,95.900452820441,-2.67111415072958));
#27906=CARTESIAN_POINT('Ctrl Pts',(-184.733319582232,96.3405488087457,-3.10349974620998));
#27907=CARTESIAN_POINT('Ctrl Pts',(-185.407131420796,95.2410911002814,-2.59999271242056));
#27908=CARTESIAN_POINT('Ctrl Pts',(-185.131072579201,95.5709154613594,-3.13562168059571));
#27909=CARTESIAN_POINT('Ctrl Pts',(-185.0456190211,96.028892389085,-3.64033156677099));
#27910=CARTESIAN_POINT('Ctrl Pts',(-185.55222076188,95.0674906005668,-2.77839835904419));
#27911=CARTESIAN_POINT('Ctrl Pts',(-185.278013603904,95.3961129331815,-3.35218099675058));
#27912=CARTESIAN_POINT('Ctrl Pts',(-185.210566100491,95.8635167264482,-3.89012301230439));
#27913=CARTESIAN_POINT('Ctrl Pts',(-185.851582277872,94.707494626045,-3.11437545164934));
#27914=CARTESIAN_POINT('Ctrl Pts',(-185.581125580994,95.0336977173119,-3.76083177968216));
#27915=CARTESIAN_POINT('Ctrl Pts',(-185.550953940504,95.5203349244564,-4.36053533295098));
#27916=CARTESIAN_POINT('Ctrl Pts',(-186.004341550726,94.5229247305643,-3.2702613765015));
#27917=CARTESIAN_POINT('Ctrl Pts',(-185.73581025216,94.8478641369735,-3.95083784102255));
#27918=CARTESIAN_POINT('Ctrl Pts',(-185.724674269717,95.344269925595,-4.57879624788273));
#27919=CARTESIAN_POINT('Ctrl Pts',(-186.468734209866,93.9589492331111,-3.71184473328433));
#27920=CARTESIAN_POINT('Ctrl Pts',(-186.206634192918,94.2793137095737,-4.49099146136749));
#27921=CARTESIAN_POINT('Ctrl Pts',(-186.252873560506,94.8059028848805,-5.19707165077033));
#27922=CARTESIAN_POINT('Ctrl Pts',(-186.786341213376,93.5694347474778,-3.97193417321456));
#27923=CARTESIAN_POINT('Ctrl Pts',(-186.528271047271,93.8870362158287,-4.81015854203247));
#27924=CARTESIAN_POINT('Ctrl Pts',(-186.614230377394,94.4335769026893,-5.56123140005082));
#27925=CARTESIAN_POINT('Ctrl Pts',(-187.429364224352,92.772219448936,-4.45009970653821));
#27926=CARTESIAN_POINT('Ctrl Pts',(-187.179275502702,93.0843625037761,-5.39983536323082));
#27927=CARTESIAN_POINT('Ctrl Pts',(-187.346070119741,93.6704353968611,-6.23072689748917));
#27928=CARTESIAN_POINT('Ctrl Pts',(-187.754922845355,92.3643571908662,-4.66770149404008));
#27929=CARTESIAN_POINT('Ctrl Pts',(-187.508904115674,92.6736124121426,-5.66953891705452));
#27930=CARTESIAN_POINT('Ctrl Pts',(-187.716714901687,93.2794672889775,-6.53539848906014));
#27931=CARTESIAN_POINT('Ctrl Pts',(-188.410112122538,91.5343223592301,-5.07270897607151));
#27932=CARTESIAN_POINT('Ctrl Pts',(-188.172164926541,91.8378317968073,-6.17425176407751));
#27933=CARTESIAN_POINT('Ctrl Pts',(-188.462886968343,92.4826689284514,-7.10246334796438));
#27934=CARTESIAN_POINT('Ctrl Pts',(-188.740497565809,91.1111729620599,-5.26033194798443));
#27935=CARTESIAN_POINT('Ctrl Pts',(-188.506622260807,91.4116871153395,-6.40936032306602));
#27936=CARTESIAN_POINT('Ctrl Pts',(-188.839274368838,92.0758984572259,-7.36516078216301));
#27937=CARTESIAN_POINT('Ctrl Pts',(-189.398843491069,90.2583421877452,-5.61022446203027));
#27938=CARTESIAN_POINT('Ctrl Pts',(-189.173011227327,90.5528941028731,-6.85041025678877));
#27939=CARTESIAN_POINT('Ctrl Pts',(-189.589532430357,91.2549207193099,-7.85505766520206));
#27940=CARTESIAN_POINT('Ctrl Pts',(-189.726873942438,89.8286042786326,-5.7725553986758));
#27941=CARTESIAN_POINT('Ctrl Pts',(-189.505024368188,90.1201178244939,-7.05626126941256));
#27942=CARTESIAN_POINT('Ctrl Pts',(-189.963481912788,90.8406631197547,-8.08234302955653));
#27943=CARTESIAN_POINT('Ctrl Pts',(-190.706530274547,88.5304660668642,-6.23019344512579));
#27944=CARTESIAN_POINT('Ctrl Pts',(-190.499557216329,88.8088485109363,-7.64207388345947));
#27945=CARTESIAN_POINT('Ctrl Pts',(-191.080632926279,89.5875778410458,-8.72309924440692));
#27946=CARTESIAN_POINT('Ctrl Pts',(-191.353674509396,87.6531907318376,-6.49656676606105));
#27947=CARTESIAN_POINT('Ctrl Pts',(-191.154383368923,87.9251930508971,-7.98648396265699));
#27948=CARTESIAN_POINT('Ctrl Pts',(-191.819082585706,88.7384854812239,-9.09605853590931));
#27949=CARTESIAN_POINT('Ctrl Pts',(-192.632970678399,85.8780091857335,-6.97723484386299));
#27950=CARTESIAN_POINT('Ctrl Pts',(-192.448889241933,86.1372754638322,-8.6170648745222));
#27951=CARTESIAN_POINT('Ctrl Pts',(-193.27977185066,87.0158621489936,-9.76906087244151));
#27952=CARTESIAN_POINT('Ctrl Pts',(-193.265161974548,84.9800606970277,-7.1911900404469));
#27953=CARTESIAN_POINT('Ctrl Pts',(-193.088386193258,85.2327644367758,-8.90204109889413));
#27954=CARTESIAN_POINT('Ctrl Pts',(-194.002055989696,86.1422915041419,-10.068628271248));
#27955=CARTESIAN_POINT('Ctrl Pts',(-195.136767560024,82.2575843111017,-7.77457663966346));
#27956=CARTESIAN_POINT('Ctrl Pts',(-194.993632951466,82.473345486734,-9.69714033640246));
#27957=CARTESIAN_POINT('Ctrl Pts',(-196.141646839768,83.4872301894655,-10.8854540504836));
#27958=CARTESIAN_POINT('Ctrl Pts',(-196.351118458959,80.4045345114431,-8.08647109199872));
#27959=CARTESIAN_POINT('Ctrl Pts',(-196.220621754019,80.6061801754008,-10.1354450942217));
#27960=CARTESIAN_POINT('Ctrl Pts',(-197.531576831738,81.6714982259837,-11.3221518808499));
#27961=CARTESIAN_POINT('Ctrl Pts',(-198.116766616771,77.5726081834688,-8.4814898062576));
#27962=CARTESIAN_POINT('Ctrl Pts',(-197.994458096547,77.7715661316189,-10.7114757703364));
#27963=CARTESIAN_POINT('Ctrl Pts',(-199.554667028181,78.8844065316243,-11.8752377009292));
#27964=CARTESIAN_POINT('Ctrl Pts',(-198.696041421195,76.6198655218917,-8.60067001276485));
#27965=CARTESIAN_POINT('Ctrl Pts',(-198.579787315131,76.8119296478313,-10.8906698919093));
#27966=CARTESIAN_POINT('Ctrl Pts',(-200.218774700134,77.9447528699897,-12.0421085545449));
#27967=CARTESIAN_POINT('Ctrl Pts',(-199.835393657519,74.6972603662356,-8.81827530517536));
#27968=CARTESIAN_POINT('Ctrl Pts',(-199.731156872596,74.8755477703346,-11.2265380697589));
#27969=CARTESIAN_POINT('Ctrl Pts',(-201.525656173084,76.0446910944109,-12.3467906967572));
#27970=CARTESIAN_POINT('Ctrl Pts',(-200.395927031185,73.7265427779827,-8.91674725157241));
#27971=CARTESIAN_POINT('Ctrl Pts',(-200.29727498786,73.8979510629713,-11.3829716214033));
#27972=CARTESIAN_POINT('Ctrl Pts',(-202.168953938337,75.0834314482927,-12.4846675143342));
#27973=CARTESIAN_POINT('Ctrl Pts',(-202.040776179842,70.8020841417172,-9.18473452855717));
#27974=CARTESIAN_POINT('Ctrl Pts',(-201.969429614348,70.9339332442469,-11.8248129171686));
#27975=CARTESIAN_POINT('Ctrl Pts',(-204.057598216847,72.1819343690171,-12.8598952638616));
#27976=CARTESIAN_POINT('Ctrl Pts',(-203.090555243157,68.8325136092258,-9.32755025230346));
#27977=CARTESIAN_POINT('Ctrl Pts',(-203.027559166486,68.9512781713152,-12.0764964747494));
#27978=CARTESIAN_POINT('Ctrl Pts',(-205.264224903837,70.2205205875485,-13.0598627591821));
#27979=CARTESIAN_POINT('Ctrl Pts',(-205.097425241471,64.8544500731044,-9.56200872917822));
#27980=CARTESIAN_POINT('Ctrl Pts',(-205.052948139998,64.9460837834979,-12.524607477045));
#27981=CARTESIAN_POINT('Ctrl Pts',(-207.572909482403,66.2457231416101,-13.3881499288596));
#27982=CARTESIAN_POINT('Ctrl Pts',(-206.054519269306,62.845953361298,-9.65350961790405));
#27983=CARTESIAN_POINT('Ctrl Pts',(-206.016439423784,62.9253694628212,-12.7190693605529));
#27984=CARTESIAN_POINT('Ctrl Pts',(-208.674970487123,64.2323356830512,-13.5162705613297));
#27985=CARTESIAN_POINT('Ctrl Pts',(-208.787453772969,56.7629489150811,-9.87162234708876));
#27986=CARTESIAN_POINT('Ctrl Pts',(-208.805906926216,56.7274477884812,-13.2469252044741));
#27987=CARTESIAN_POINT('Ctrl Pts',(-211.824237457266,58.1168549195064,-13.8216808903116));
#27988=CARTESIAN_POINT('Ctrl Pts',(-210.425226591334,52.631005892894,-9.94272536792823));
#27989=CARTESIAN_POINT('Ctrl Pts',(-210.440269997768,52.5822843956569,-13.5057475829278));
#27990=CARTESIAN_POINT('Ctrl Pts',(-213.714800431993,53.9395725306549,-13.9212498502496));
#27991=CARTESIAN_POINT('Ctrl Pts',(-212.604000467011,46.3190573027775,-9.9921716805904));
#27992=CARTESIAN_POINT('Ctrl Pts',(-212.606234394252,46.3108044017127,-13.8219499339134));
#27993=CARTESIAN_POINT('Ctrl Pts',(-216.232554404446,47.5307358639797,-13.9905049124008));
#27994=CARTESIAN_POINT('Ctrl Pts',(-213.283880548139,44.1960440918465,-9.99883242576813));
#27995=CARTESIAN_POINT('Ctrl Pts',(-213.287229079501,44.1810847215626,-13.9153550243481));
#27996=CARTESIAN_POINT('Ctrl Pts',(-217.018726572062,45.370602602594,-13.9998386774369));
#27997=CARTESIAN_POINT('Ctrl Pts',(-214.549838598837,39.9117037182066,-9.99904891274098));
#27998=CARTESIAN_POINT('Ctrl Pts',(-214.55760511708,39.8815809871525,-14.082597114446));
#27999=CARTESIAN_POINT('Ctrl Pts',(-218.483320257025,41.0034462363903,-14.0001571760684));
#28000=CARTESIAN_POINT('Ctrl Pts',(-215.136376568597,37.7485084112375,-9.99258580907847));
#28001=CARTESIAN_POINT('Ctrl Pts',(-215.143908548574,37.7144923110325,-14.1558384825482));
#28002=CARTESIAN_POINT('Ctrl Pts',(-219.162273921736,38.7945126487825,-13.991115461238));
#28003=CARTESIAN_POINT('Ctrl Pts',(-216.749953158185,31.2125703645965,-9.96182675340658));
#28004=CARTESIAN_POINT('Ctrl Pts',(-216.775802051944,31.100378487788,-14.3531964080252));
#28005=CARTESIAN_POINT('Ctrl Pts',(-221.030846972258,32.1103382810994,-13.9480701212897));
#28006=CARTESIAN_POINT('Ctrl Pts',(-217.620747415908,26.8377335828005,-9.92696743661106));
#28007=CARTESIAN_POINT('Ctrl Pts',(-217.634052712766,26.7487700574455,-14.4478056294438));
#28008=CARTESIAN_POINT('Ctrl Pts',(-222.040310058227,27.6230828990521,-13.899275220772));
#28009=CARTESIAN_POINT('Ctrl Pts',(-218.964732221164,18.0539614072054,-9.86263998637371));
#28010=CARTESIAN_POINT('Ctrl Pts',(-218.976069418789,17.9643982345151,-14.5927859676098));
#28011=CARTESIAN_POINT('Ctrl Pts',(-223.598907254315,18.5974327804109,-13.8092287551284));
#28012=CARTESIAN_POINT('Ctrl Pts',(-219.437897325133,13.6450084731965,-9.83311006111365));
#28013=CARTESIAN_POINT('Ctrl Pts',(-219.440263256372,13.5936991145387,-14.6404855064752));
#28014=CARTESIAN_POINT('Ctrl Pts',(-224.148014046288,14.0590074436304,-13.7678907295765));
#28015=CARTESIAN_POINT('Ctrl Pts',(-219.988849745161,4.79313733566884,-9.79797610395582));
#28016=CARTESIAN_POINT('Ctrl Pts',(-219.98909361829,4.7573196656202,-14.6968909906386));
#28017=CARTESIAN_POINT('Ctrl Pts',(-224.787432850351,4.94061146060701,-13.7187075789802));
#28018=CARTESIAN_POINT('Ctrl Pts',(-220.066648600991,0.350203291743644,
-9.79239486915522));
#28019=CARTESIAN_POINT('Ctrl Pts',(-220.065259345099,0.361024215332044,
-14.7045472577049));
#28020=CARTESIAN_POINT('Ctrl Pts',(-224.877757641866,0.360614518566908,
-13.7108944521662));
#28021=CARTESIAN_POINT('Ctrl Pts',(-219.881289785246,-6.34015037874837,
-9.80469728794968));
#28022=CARTESIAN_POINT('Ctrl Pts',(-219.880459455254,-6.32388335486397,
-14.6856874469098));
#28023=CARTESIAN_POINT('Ctrl Pts',(-224.662609304112,-6.53393892017589,
-13.7281163920661));
#28024=CARTESIAN_POINT('Ctrl Pts',(-219.7690846214,-8.5746040811491,-9.81212397201967));
#28025=CARTESIAN_POINT('Ctrl Pts',(-219.769195818231,-8.54934036973086,
-14.6743297915045));
#28026=CARTESIAN_POINT('Ctrl Pts',(-224.53237253079,-8.83622233241281,-13.7385128649179));
#28027=CARTESIAN_POINT('Ctrl Pts',(-219.441946243719,-13.0523359205035,
-9.83258686591823));
#28028=CARTESIAN_POINT('Ctrl Pts',(-219.443263597349,-13.0197708223219,
-14.6407181348838));
#28029=CARTESIAN_POINT('Ctrl Pts',(-224.152727496901,-13.4479084088541,
-13.767158287495));
#28030=CARTESIAN_POINT('Ctrl Pts',(-219.228078485099,-15.2805016753907,
-9.84554939701803));
#28031=CARTESIAN_POINT('Ctrl Pts',(-219.230954294149,-15.2408197429134,
-14.6187137573007));
#28032=CARTESIAN_POINT('Ctrl Pts',(-223.904556238525,-15.7417406054664,
-13.7853040799473));
#28033=CARTESIAN_POINT('Ctrl Pts',(-218.439133922489,-21.9259584225567,
-9.88922199339624));
#28034=CARTESIAN_POINT('Ctrl Pts',(-218.44812769664,-21.846612569119,-14.5362234536541));
#28035=CARTESIAN_POINT('Ctrl Pts',(-222.98929920683,-22.5783142290943,-13.8464389966528));
#28036=CARTESIAN_POINT('Ctrl Pts',(-217.716767444137,-26.3076453874502,
-9.92513263870734));
#28037=CARTESIAN_POINT('Ctrl Pts',(-217.737140154904,-26.2008567667317,
-14.460378345458));
#28038=CARTESIAN_POINT('Ctrl Pts',(-222.151504324182,-27.0796752766318,
-13.8967075271592));
#28039=CARTESIAN_POINT('Ctrl Pts',(-215.887601531786,-34.9758113643062,
-9.98260158823235));
#28040=CARTESIAN_POINT('Ctrl Pts',(-215.90681504924,-34.8830703988305,-14.2500621399759));
#28041=CARTESIAN_POINT('Ctrl Pts',(-220.03196646784,-35.9627273160852,-13.9771458586264));
#28042=CARTESIAN_POINT('Ctrl Pts',(-214.780781254865,-39.262299527481,-10.004263728387));
#28043=CARTESIAN_POINT('Ctrl Pts',(-214.811197566452,-39.1599104852413,
-14.1192077667389));
#28044=CARTESIAN_POINT('Ctrl Pts',(-218.750199620032,-40.344439125031,-14.007461154831));
#28045=CARTESIAN_POINT('Ctrl Pts',(-212.181660240525,-47.739771588893,-9.99138531231972));
#28046=CARTESIAN_POINT('Ctrl Pts',(-212.20113399609,-47.6723891640227,-13.7680488609868));
#28047=CARTESIAN_POINT('Ctrl Pts',(-215.743991965115,-48.9786473240517,
-13.9893987794769));
#28048=CARTESIAN_POINT('Ctrl Pts',(-210.689374656748,-51.9307717632098,
-9.95731215039984));
#28049=CARTESIAN_POINT('Ctrl Pts',(-210.715881161589,-51.8691066101861,
-13.5540230017111));
#28050=CARTESIAN_POINT('Ctrl Pts',(-214.019565211694,-53.2311754970819,
-13.9416762189794));
#28051=CARTESIAN_POINT('Ctrl Pts',(-208.153987483228,-58.143634952563,-9.81667719355973));
#28052=CARTESIAN_POINT('Ctrl Pts',(-208.131332303436,-58.1943415635481,
-13.1152950231644));
#28053=CARTESIAN_POINT('Ctrl Pts',(-211.0944995106,-59.5034442639553,-13.7447444436423));
#28054=CARTESIAN_POINT('Ctrl Pts',(-207.257503549638,-60.2058166920358,
-9.75447716181983));
#28055=CARTESIAN_POINT('Ctrl Pts',(-207.229900666133,-60.2678296059469,
-12.9529654277891));
#28056=CARTESIAN_POINT('Ctrl Pts',(-210.060944633878,-61.5799263735734,
-13.657648433114));
#28057=CARTESIAN_POINT('Ctrl Pts',(-205.378237956305,-64.273628314509,-9.58938880230249));
#28058=CARTESIAN_POINT('Ctrl Pts',(-205.334959986084,-64.3617609972516,
-12.5816370076419));
#28059=CARTESIAN_POINT('Ctrl Pts',(-207.896217583744,-65.663879283607,-13.4264876763358));
#28060=CARTESIAN_POINT('Ctrl Pts',(-204.394451399662,-66.2821759898736,
-9.48655954038466));
#28061=CARTESIAN_POINT('Ctrl Pts',(-204.344150257108,-66.3831240343329,
-12.3740275121672));
#28062=CARTESIAN_POINT('Ctrl Pts',(-206.763884251522,-67.6743142351468,
-13.2825059299792));
#28063=CARTESIAN_POINT('Ctrl Pts',(-202.339871295312,-70.2481208611195,
-9.22591917108276));
#28064=CARTESIAN_POINT('Ctrl Pts',(-202.270084276028,-70.3765254341986,
-11.8962907953015));
#28065=CARTESIAN_POINT('Ctrl Pts',(-204.401337671746,-71.6306725650387,
-12.9175609319477));
#28066=CARTESIAN_POINT('Ctrl Pts',(-201.269068012198,-72.2055260456701,
-9.06826451525565));
#28067=CARTESIAN_POINT('Ctrl Pts',(-201.190292857267,-72.347448988328,-11.6282123344199));
#28068=CARTESIAN_POINT('Ctrl Pts',(-203.171113874487,-73.5766035176501,
-12.6968171747456));
#28069=CARTESIAN_POINT('Ctrl Pts',(-199.041608375758,-76.068143900156,-8.67680213528545));
#28070=CARTESIAN_POINT('Ctrl Pts',(-198.939568678494,-76.2380118061437,
-11.0054857284394));
#28071=CARTESIAN_POINT('Ctrl Pts',(-200.614737956183,-77.4019017685666,
-12.1487056946224));
#28072=CARTESIAN_POINT('Ctrl Pts',(-197.884929568798,-77.9733779132744,
-8.44340949232921));
#28073=CARTESIAN_POINT('Ctrl Pts',(-197.771960106038,-78.1570310417782,
-10.6538744553092));
#28074=CARTESIAN_POINT('Ctrl Pts',(-199.288560854474,-79.2812891203015,
-11.8219197811625));
#28075=CARTESIAN_POINT('Ctrl Pts',(-196.086592698953,-80.7905481256368,
-8.00941122339776));
#28076=CARTESIAN_POINT('Ctrl Pts',(-195.942000534272,-81.0127720267323,
-10.0264388695469));
#28077=CARTESIAN_POINT('Ctrl Pts',(-197.229092539617,-82.0481576896257,
-11.2142562418261));
#28078=CARTESIAN_POINT('Ctrl Pts',(-195.476435527691,-81.7229977482265,
-7.85053630037284));
#28079=CARTESIAN_POINT('Ctrl Pts',(-195.325118084347,-81.9520318404096,
-9.80294658045898));
#28080=CARTESIAN_POINT('Ctrl Pts',(-196.530724565999,-82.9619066522144,
-10.9918079629887));
#28081=CARTESIAN_POINT('Ctrl Pts',(-194.240854639226,-83.5658540109184,
-7.49863854644174));
#28082=CARTESIAN_POINT('Ctrl Pts',(-194.075388956764,-83.8082449326526,
-9.31739070142719));
#28083=CARTESIAN_POINT('Ctrl Pts',(-195.117357931181,-84.7635976184135,
-10.499100026407));
#28084=CARTESIAN_POINT('Ctrl Pts',(-193.614824846021,-84.4772228383163,
-7.30555596453726));
#28085=CARTESIAN_POINT('Ctrl Pts',(-193.442219094693,-84.7263031125253,
-9.05574333461493));
#28086=CARTESIAN_POINT('Ctrl Pts',(-194.401665096834,-85.6524857281427,
-10.22875684803));
#28087=CARTESIAN_POINT('Ctrl Pts',(-192.347932759001,-86.2784285351058,
-6.87464479646914));
#28088=CARTESIAN_POINT('Ctrl Pts',(-192.160442100619,-86.5404947454048,
-8.48135963635239));
#28089=CARTESIAN_POINT('Ctrl Pts',(-192.954216968456,-87.4049400733434,
-9.62542037310025));
#28090=CARTESIAN_POINT('Ctrl Pts',(-191.707044521612,-87.1682928180243,
-6.63700210622506));
#28091=CARTESIAN_POINT('Ctrl Pts',(-191.512033111158,-87.4368721369655,
-8.16951011355977));
#28092=CARTESIAN_POINT('Ctrl Pts',(-192.222432355974,-88.2685319889458,
-9.29268753771301));
#28093=CARTESIAN_POINT('Ctrl Pts',(-190.378144990072,-88.9713989982768,
-6.08509931817266));
#28094=CARTESIAN_POINT('Ctrl Pts',(-190.167610974008,-89.2522458880518,
-7.45565276123948));
#28095=CARTESIAN_POINT('Ctrl Pts',(-190.706025517156,-90.0138628646082,
-8.51994753802441));
#28096=CARTESIAN_POINT('Ctrl Pts',(-189.689332036395,-89.8834557429178,
-5.76804029795621));
#28097=CARTESIAN_POINT('Ctrl Pts',(-189.470454598868,-90.1710185021602,
-7.05122460308101));
#28098=CARTESIAN_POINT('Ctrl Pts',(-189.920463440167,-90.8942884726876,
-8.07597136681174));
#28099=CARTESIAN_POINT('Ctrl Pts',(-188.996710505551,-90.7791921163431,
-5.39631620992176));
#28100=CARTESIAN_POINT('Ctrl Pts',(-188.764974135119,-91.0786621249365,
-6.58013865011089));
#28101=CARTESIAN_POINT('Ctrl Pts',(-189.131271676234,-91.7562941904943,
-7.55556514077405));
#28102=CARTESIAN_POINT('',(-189.102923332965,-90.6416650378459,-5.4533811546917));
#28103=CARTESIAN_POINT('',(-188.850942384682,90.9673968784445,5.31766757924549));
#28104=CARTESIAN_POINT('Ctrl Pts',(-189.102923332965,-90.641665037846,-5.4533811546917));
#28105=CARTESIAN_POINT('Ctrl Pts',(-189.582260717675,-90.020253446221,-5.70696955389192));
#28106=CARTESIAN_POINT('Ctrl Pts',(-190.058170492541,-89.3930857113232,
-5.93411277433641));
#28107=CARTESIAN_POINT('Ctrl Pts',(-190.53003087708,-88.7608183026999,-6.14212704225141));
#28108=CARTESIAN_POINT('Ctrl Pts',(-190.710986586798,-88.5183474333337,
-6.22189930268113));
#28109=CARTESIAN_POINT('Ctrl Pts',(-190.891347174418,-88.2751269204779,
-6.29885831045948));
#28110=CARTESIAN_POINT('Ctrl Pts',(-191.071079133441,-88.0311950960934,
-6.37341669810158));
#28111=CARTESIAN_POINT('Ctrl Pts',(-191.646252706304,-87.250570772353,-6.61201652442255));
#28112=CARTESIAN_POINT('Ctrl Pts',(-192.215025141179,-86.4626063253748,
-6.82549480142756));
#28113=CARTESIAN_POINT('Ctrl Pts',(-192.776838225234,-85.6678937138362,
-7.02043059393256));
#28114=CARTESIAN_POINT('Ctrl Pts',(-192.848364962895,-85.566715578091,-7.04524867255532));
#28115=CARTESIAN_POINT('Ctrl Pts',(-192.919778950195,-85.4654281068113,
-7.06976619818262));
#28116=CARTESIAN_POINT('Ctrl Pts',(-192.991079081859,-85.36403256041,-7.09399674750343));
#28117=CARTESIAN_POINT('Ctrl Pts',(-193.713446564455,-84.3367575205096,
-7.33948522706467));
#28118=CARTESIAN_POINT('Ctrl Pts',(-194.424096824214,-83.2984253835442,
-7.55590148935084));
#28119=CARTESIAN_POINT('Ctrl Pts',(-195.122436963889,-82.2496188764938,
-7.74993375843261));
#28120=CARTESIAN_POINT('Ctrl Pts',(-195.644764721679,-81.4651576661762,
-7.89506137503431));
#28121=CARTESIAN_POINT('Ctrl Pts',(-196.160206469516,-80.6748374593551,
-8.02766652837252));
#28122=CARTESIAN_POINT('Ctrl Pts',(-196.668528283489,-79.8789148564568,
-8.15054780740364));
#28123=CARTESIAN_POINT('Ctrl Pts',(-197.685784336456,-78.2861107248307,
-8.39645841256492));
#28124=CARTESIAN_POINT('Ctrl Pts',(-198.674593142452,-76.6707691018819,
-8.60245660480754));
#28125=CARTESIAN_POINT('Ctrl Pts',(-199.633903813475,-75.03378970395,-8.77941525971185));
#28126=CARTESIAN_POINT('Ctrl Pts',(-199.794861726751,-74.7591291628693,
-8.80910626252247));
#28127=CARTESIAN_POINT('Ctrl Pts',(-199.954989254821,-74.4838595913707,
-8.83797975018607));
#28128=CARTESIAN_POINT('Ctrl Pts',(-200.114281483532,-74.2079853746882,
-8.8660870801691));
#28129=CARTESIAN_POINT('Ctrl Pts',(-201.031953371716,-72.6186924419847,
-9.02801153050877));
#28130=CARTESIAN_POINT('Ctrl Pts',(-201.921922786274,-71.0093050648385,
-9.16424853724766));
#28131=CARTESIAN_POINT('Ctrl Pts',(-202.783481319878,-69.3802201617152,
-9.28065045514811));
#28132=CARTESIAN_POINT('Ctrl Pts',(-202.962805445657,-69.0411436919492,
-9.30487826016919));
#28133=CARTESIAN_POINT('Ctrl Pts',(-203.140898579713,-68.701213916756,-9.32824677071867));
#28134=CARTESIAN_POINT('Ctrl Pts',(-203.317754052504,-68.3604344681444,
-9.35080875744684));
#28135=CARTESIAN_POINT('Ctrl Pts',(-204.055553774916,-66.9387822081274,
-9.44493209602629));
#28136=CARTESIAN_POINT('Ctrl Pts',(-204.771821585756,-65.5023355039341,
-9.52494371021979));
#28137=CARTESIAN_POINT('Ctrl Pts',(-205.466126479309,-64.0511971714295,
-9.59344287612378));
#28138=CARTESIAN_POINT('Ctrl Pts',(-205.737857546834,-63.4832631529902,
-9.62025148952761));
#28139=CARTESIAN_POINT('Ctrl Pts',(-206.006223960639,-62.9130787823288,
-9.64529672325964));
#28140=CARTESIAN_POINT('Ctrl Pts',(-206.271197699333,-62.340650239919,-9.66873439603508));
#28141=CARTESIAN_POINT('Ctrl Pts',(-206.584024550177,-61.6648435764407,
-9.69640481123029));
#28142=CARTESIAN_POINT('Ctrl Pts',(-206.892247081492,-60.9856295693903,
-9.72182534319836));
#28143=CARTESIAN_POINT('Ctrl Pts',(-207.195451326658,-60.3038399562509,
-9.74517566651772));
#28144=CARTESIAN_POINT('Ctrl Pts',(-207.500367398821,-59.6182011032537,
-9.76865782082053));
#28145=CARTESIAN_POINT('Ctrl Pts',(-207.800208254404,-58.9299575759062,
-9.79004632456711));
#28146=CARTESIAN_POINT('Ctrl Pts',(-208.094601304795,-58.239977290383,-9.80952391276348));
#28147=CARTESIAN_POINT('Ctrl Pts',(-208.388994355186,-57.5499970048598,
-9.82900150095984));
#28148=CARTESIAN_POINT('Ctrl Pts',(-208.677939560999,-56.8582800885254,
-9.846568173606));
#28149=CARTESIAN_POINT('Ctrl Pts',(-208.961113653817,-56.1657146913821,
-9.86240666570794));
#28150=CARTESIAN_POINT('Ctrl Pts',(-209.495139736396,-54.8596348085616,
-9.89227581018714));
#28151=CARTESIAN_POINT('Ctrl Pts',(-210.009433697182,-53.5486516972336,
-9.9161782204413));
#28152=CARTESIAN_POINT('Ctrl Pts',(-210.504209260612,-52.2328373293754,
-9.93512269107262));
#28153=CARTESIAN_POINT('Ctrl Pts',(-211.00063112145,-50.9126447707905,-9.95413019681563));
#28154=CARTESIAN_POINT('Ctrl Pts',(-211.477404605655,-49.5875884934105,
-9.96814671432499));
#28155=CARTESIAN_POINT('Ctrl Pts',(-211.934701650502,-48.2577123828032,
-9.97819114162064));
#28156=CARTESIAN_POINT('Ctrl Pts',(-212.393661440177,-46.9230008055126,
-9.98827209073449));
#28157=CARTESIAN_POINT('Ctrl Pts',(-212.833003021567,-45.583434018586,-9.99435201185891));
#28158=CARTESIAN_POINT('Ctrl Pts',(-213.252854163575,-44.2390313383672,
-9.99746095769943));
#28159=CARTESIAN_POINT('Ctrl Pts',(-213.321782825185,-44.0183153079917,
-9.9979713659236));
#28160=CARTESIAN_POINT('Ctrl Pts',(-213.390186056062,-43.797468885728,-9.99840169710009));
#28161=CARTESIAN_POINT('Ctrl Pts',(-213.45806430009,-43.5764921004782,-9.99875650921472));
#28162=CARTESIAN_POINT('Ctrl Pts',(-213.878746211512,-42.2069673325635,
-10.0009554912408));
#28163=CARTESIAN_POINT('Ctrl Pts',(-214.279264487762,-40.8324457380546,
-10.0002042865536));
#28164=CARTESIAN_POINT('Ctrl Pts',(-214.659689264104,-39.4529486973177,
-9.9972139224554));
#28165=CARTESIAN_POINT('Ctrl Pts',(-215.059027314902,-38.0048683051126,
-9.99407488881614));
#28166=CARTESIAN_POINT('Ctrl Pts',(-215.436224812888,-36.5513052574736,
-9.98846851623776));
#28167=CARTESIAN_POINT('Ctrl Pts',(-215.791304305115,-35.0922648472616,
-9.98121724046361));
#28168=CARTESIAN_POINT('Ctrl Pts',(-216.146383797341,-33.6332244370496,
-9.97396596468947));
#28169=CARTESIAN_POINT('Ctrl Pts',(-216.479345374389,-32.1687062920674,
-9.96506978571955));
#28170=CARTESIAN_POINT('Ctrl Pts',(-216.79015016326,-30.6987012818522,-9.95535113929721));
#28171=CARTESIAN_POINT('Ctrl Pts',(-217.083045980536,-29.3133998505938,
-9.94619249377886));
#28172=CARTESIAN_POINT('Ctrl Pts',(-217.356262700494,-27.9232340571749,
-9.93629265774494));
#28173=CARTESIAN_POINT('Ctrl Pts',(-217.609720097247,-26.5281727798487,
-9.92610877818971));
#28174=CARTESIAN_POINT('Ctrl Pts',(-217.862641171742,-25.1360634874478,
-9.91594644798103));
#28175=CARTESIAN_POINT('Ctrl Pts',(-218.095886491803,-23.7390791164929,
-9.90550127506577));
#28176=CARTESIAN_POINT('Ctrl Pts',(-218.309324573698,-22.3371857234748,
-9.8952275105708));
#28177=CARTESIAN_POINT('Ctrl Pts',(-218.521921535319,-20.9408169348002,
-9.88499423309448));
#28178=CARTESIAN_POINT('Ctrl Pts',(-218.714867074954,-19.5395774505493,
-9.87493101572222));
#28179=CARTESIAN_POINT('Ctrl Pts',(-218.887979530425,-18.1334350540361,
-9.86548676035596));
#28180=CARTESIAN_POINT('Ctrl Pts',(-218.912596242757,-17.9334806210731,
-9.86414378063271));
#28181=CARTESIAN_POINT('Ctrl Pts',(-218.936811823662,-17.7334270525466,
-9.86281331696435));
#28182=CARTESIAN_POINT('Ctrl Pts',(-218.960625665239,-17.5332742632934,
-9.86149666014403));
#28183=CARTESIAN_POINT('Ctrl Pts',(-219.184812192997,-15.6490104959437,
-9.84910148568848));
#28184=CARTESIAN_POINT('Ctrl Pts',(-219.373454863963,-13.7554245499718,
-9.83785494815097));
#28185=CARTESIAN_POINT('Ctrl Pts',(-219.525841126991,-11.8536894372336,
-9.82845661547209));
#28186=CARTESIAN_POINT('Ctrl Pts',(-219.552867756293,-11.5164051643565,
-9.82678976408852));
#28187=CARTESIAN_POINT('Ctrl Pts',(-219.578753985703,-11.1788646797448,
-9.8251810483157));
#28188=CARTESIAN_POINT('Ctrl Pts',(-219.603495908495,-10.8410746855513,
-9.82363437087996));
#28189=CARTESIAN_POINT('Ctrl Pts',(-219.705373439927,-9.45018800954576,
-9.81726575998433));
#28190=CARTESIAN_POINT('Ctrl Pts',(-219.787419394757,-8.06100294968608,
-9.81197810113728));
#28191=CARTESIAN_POINT('Ctrl Pts',(-219.849875987437,-6.6735051628098,-9.80789674793111));
#28192=CARTESIAN_POINT('Ctrl Pts',(-219.888111421962,-5.82408993686036,
-9.80539817561728));
#28193=CARTESIAN_POINT('Ctrl Pts',(-219.919004199351,-4.97530671931527,
-9.80335170157182));
#28194=CARTESIAN_POINT('Ctrl Pts',(-219.942600668612,-4.12714946555835,
-9.80178608653178));
#28195=CARTESIAN_POINT('Ctrl Pts',(-219.982142675654,-2.70584190766221,
-9.79916249228756));
#28196=CARTESIAN_POINT('Ctrl Pts',(-220.001198185544,-1.28628743268108,
-9.79793805992874));
#28197=CARTESIAN_POINT('Ctrl Pts',(-219.999941724939,0.131516457556867,
-9.79805476787017));
#28198=CARTESIAN_POINT('Ctrl Pts',(-219.998682147343,1.55283759632288,-9.79817176533743));
#28199=CARTESIAN_POINT('Ctrl Pts',(-219.977009716239,2.97239974751487,-9.79963656548587));
#28200=CARTESIAN_POINT('Ctrl Pts',(-219.935048547014,4.3902139918877,-9.80239071384323));
#28201=CARTESIAN_POINT('Ctrl Pts',(-219.892987902636,5.81138937446998,-9.80515139131631));
#28202=CARTESIAN_POINT('Ctrl Pts',(-219.830542222622,7.23080884893533,-9.80920753742537));
#28203=CARTESIAN_POINT('Ctrl Pts',(-219.74778437218,8.64848773576876,-9.81450028098692));
#28204=CARTESIAN_POINT('Ctrl Pts',(-219.736609773761,8.83991359037877,-9.81521494773474));
#28205=CARTESIAN_POINT('Ctrl Pts',(-219.725064756642,9.03130771205525,-9.81595216070532));
#28206=CARTESIAN_POINT('Ctrl Pts',(-219.713149427464,9.22267013971849,-9.81671177496444));
#28207=CARTESIAN_POINT('Ctrl Pts',(-219.624287664256,10.6498067701466,-9.82237680204124));
#28208=CARTESIAN_POINT('Ctrl Pts',(-219.514834598448,12.0751717546752,-9.82928536128041));
#28209=CARTESIAN_POINT('Ctrl Pts',(-219.38480626819,13.4987695466866,-9.83712441968859));
#28210=CARTESIAN_POINT('Ctrl Pts',(-219.254821792827,14.9218871992416,-9.84496083420306));
#28211=CARTESIAN_POINT('Ctrl Pts',(-219.104275899337,16.3432391502397,-9.85372712033006));
#28212=CARTESIAN_POINT('Ctrl Pts',(-218.933132808931,17.7628245558423,-9.86311056170108));
#28213=CARTESIAN_POINT('Ctrl Pts',(-218.762257656336,19.1801874901504,-9.87247931256528));
#28214=CARTESIAN_POINT('Ctrl Pts',(-218.570849700195,20.5957897010906,-9.88246328777715));
#28215=CARTESIAN_POINT('Ctrl Pts',(-218.358822292918,22.0096206245496,-9.89275123741531));
#28216=CARTESIAN_POINT('Ctrl Pts',(-218.335813724675,22.1630452487734,-9.89386765436523));
#28217=CARTESIAN_POINT('Ctrl Pts',(-218.312562294107,22.3164490024472,-9.89498765089645));
#28218=CARTESIAN_POINT('Ctrl Pts',(-218.289067854669,22.4698318628755,-9.89611082926645));
#28219=CARTESIAN_POINT('Ctrl Pts',(-218.077188114775,23.8530834470226,-9.90623998095426));
#28220=CARTESIAN_POINT('Ctrl Pts',(-217.845550020112,25.2346280157213,-9.91663409193066));
#28221=CARTESIAN_POINT('Ctrl Pts',(-217.594014743781,26.6144719940167,-9.92675978258888));
#28222=CARTESIAN_POINT('Ctrl Pts',(-217.343223872589,27.9902323981778,-9.93685550680951));
#28223=CARTESIAN_POINT('Ctrl Pts',(-217.072653340494,29.3643025370337,-9.94668439711208));
#28224=CARTESIAN_POINT('Ctrl Pts',(-216.782117050876,30.736670744236,-9.955717795414));
#28225=CARTESIAN_POINT('Ctrl Pts',(-216.493058233207,32.1020600107562,-9.96470525593437));
#28226=CARTESIAN_POINT('Ctrl Pts',(-216.184236108853,33.4657648725542,-9.97290529455565));
#28227=CARTESIAN_POINT('Ctrl Pts',(-215.855420636239,34.8277519779683,-9.97979727744779));
#28228=CARTESIAN_POINT('Ctrl Pts',(-215.792138141171,35.0898745040037,-9.98112368058178));
#28229=CARTESIAN_POINT('Ctrl Pts',(-215.728114969485,35.3519333335032,-9.98240163425538));
#28230=CARTESIAN_POINT('Ctrl Pts',(-215.663349285992,35.6139281225462,-9.98362742716542));
#28231=CARTESIAN_POINT('Ctrl Pts',(-215.378618518289,36.7657414501431,-9.98901640690739));
#28232=CARTESIAN_POINT('Ctrl Pts',(-215.080318928169,37.9131343588526,-9.9933404843776));
#28233=CARTESIAN_POINT('Ctrl Pts',(-214.768739822526,39.0553552393069,-9.99618853751749));
#28234=CARTESIAN_POINT('Ctrl Pts',(-214.490069922121,40.0769339434976,-9.99873577727286));
#28235=CARTESIAN_POINT('Ctrl Pts',(-214.200778251147,41.094375598618,-10.0001023240286));
#28236=CARTESIAN_POINT('Ctrl Pts',(-213.901104808522,42.1071550347656,-9.99999405004369));
#28237=CARTESIAN_POINT('Ctrl Pts',(-213.492922283981,43.4866528755784,-9.99984657101419));
#28238=CARTESIAN_POINT('Ctrl Pts',(-213.065281545394,44.8581999124421,-9.99697039599626));
#28239=CARTESIAN_POINT('Ctrl Pts',(-212.618337105391,46.2218293651797,-9.99049076100407));
#28240=CARTESIAN_POINT('Ctrl Pts',(-212.370269085231,46.9786859860388,-9.98689436270485));
#28241=CARTESIAN_POINT('Ctrl Pts',(-212.116253451429,47.733103416628,-9.98218788464245));
#28242=CARTESIAN_POINT('Ctrl Pts',(-211.856309787049,48.4850862480963,-9.97622175746237));
#28243=CARTESIAN_POINT('Ctrl Pts',(-211.379488601213,49.8644672239142,-9.96527794067941));
#28244=CARTESIAN_POINT('Ctrl Pts',(-210.882722773809,51.2356606005683,-9.95022000519016));
#28245=CARTESIAN_POINT('Ctrl Pts',(-210.36610102331,52.5986610272489,-9.92976988604603));
#28246=CARTESIAN_POINT('Ctrl Pts',(-209.835337069147,53.9989727549137,-9.9087599574289));
#28247=CARTESIAN_POINT('Ctrl Pts',(-209.283615347521,55.3906372337196,-9.88205858904313));
#28248=CARTESIAN_POINT('Ctrl Pts',(-208.710977413956,56.7736317201052,-9.84827985780893));
#28249=CARTESIAN_POINT('Ctrl Pts',(-208.138339480391,58.1566262064908,-9.81450112657472));
#28250=CARTESIAN_POINT('Ctrl Pts',(-207.54478519928,59.5309510279822,-9.77364503249207));
#28251=CARTESIAN_POINT('Ctrl Pts',(-206.930302679868,60.8965613623573,-9.72432565248121));
#28252=CARTESIAN_POINT('Ctrl Pts',(-206.32754650778,62.2361113604596,-9.67594744843798));
#28253=CARTESIAN_POINT('Ctrl Pts',(-205.704653571512,63.5672747476244,-9.61968076721895));
#28254=CARTESIAN_POINT('Ctrl Pts',(-205.061572025718,64.8899703091143,-9.55306338132051));
#28255=CARTESIAN_POINT('Ctrl Pts',(-204.408458319862,66.2333001022554,-9.48540675509146));
#28256=CARTESIAN_POINT('Ctrl Pts',(-203.734521172266,67.5678961860887,-9.40707396037423));
#28257=CARTESIAN_POINT('Ctrl Pts',(-203.039660016423,68.8936434234688,-9.31548572940536));
#28258=CARTESIAN_POINT('Ctrl Pts',(-202.34479886058,70.2193906608489,-9.22389749843649));
#28259=CARTESIAN_POINT('Ctrl Pts',(-201.629013533948,71.5362893553416,-9.11905383121599));
#28260=CARTESIAN_POINT('Ctrl Pts',(-200.892159193484,72.8441895279559,-8.99837545998041));
#28261=CARTESIAN_POINT('Ctrl Pts',(-200.586970936635,73.3858919403522,-8.94839323183244));
#28262=CARTESIAN_POINT('Ctrl Pts',(-200.278025369755,73.9262941980819,-8.89557299390327));
#28263=CARTESIAN_POINT('Ctrl Pts',(-199.965848931004,74.4644603316202,-8.83971192769632));
#28264=CARTESIAN_POINT('Ctrl Pts',(-199.715624687529,74.8958260495664,-8.79493662983211));
#28265=CARTESIAN_POINT('Ctrl Pts',(-199.463325568433,75.3257555676997,-8.7482076655061));
#28266=CARTESIAN_POINT('Ctrl Pts',(-199.209243550892,75.7537790987561,-8.69942058786797));
#28267=CARTESIAN_POINT('Ctrl Pts',(-198.638172186973,76.7157990954304,-8.5897674009244));
#28268=CARTESIAN_POINT('Ctrl Pts',(-198.057534390405,77.6691493924228,-8.46965732294354));
#28269=CARTESIAN_POINT('Ctrl Pts',(-197.467674066489,78.6136055049731,-8.33695469259649));
#28270=CARTESIAN_POINT('Ctrl Pts',(-196.830489808791,79.6338344347796,-8.19360545620275));
#28271=CARTESIAN_POINT('Ctrl Pts',(-196.182500603122,80.6437484421905,-8.03598349849812));
#28272=CARTESIAN_POINT('Ctrl Pts',(-195.524339684909,81.6427983389507,-7.85954724113827));
#28273=CARTESIAN_POINT('Ctrl Pts',(-194.963942524463,82.4934485519824,-7.70931896886041));
#28274=CARTESIAN_POINT('Ctrl Pts',(-194.39617173317,83.3362230411495,-7.54545065392799));
#28275=CARTESIAN_POINT('Ctrl Pts',(-193.821438603718,84.1708044967981,-7.36513881081726));
#28276=CARTESIAN_POINT('Ctrl Pts',(-193.278404315604,84.9593554318606,-7.19477189033818));
#28277=CARTESIAN_POINT('Ctrl Pts',(-192.729171431316,85.7405634546523,-7.00954588434748));
#28278=CARTESIAN_POINT('Ctrl Pts',(-192.174344836506,86.5138551176446,-6.8048710633828));
#28279=CARTESIAN_POINT('Ctrl Pts',(-192.090736617309,86.6303843890734,-6.7740280982918));
#28280=CARTESIAN_POINT('Ctrl Pts',(-192.007001446041,86.7467339588819,-6.74274348491311));
#28281=CARTESIAN_POINT('Ctrl Pts',(-191.923141467766,86.862901934308,-6.71100151736954));
#28282=CARTESIAN_POINT('Ctrl Pts',(-191.455364919845,87.5108946436029,-6.53394270687155));
#28283=CARTESIAN_POINT('Ctrl Pts',(-190.983682123568,88.1532614843595,-6.34284056508145));
#28284=CARTESIAN_POINT('Ctrl Pts',(-190.508729882859,88.7893533408363,-6.13265396746052));
#28285=CARTESIAN_POINT('Ctrl Pts',(-190.333501788842,89.0240320181371,-6.05510807182643));
#28286=CARTESIAN_POINT('Ctrl Pts',(-190.157829060128,89.2578569081404,-5.97496448588751));
#28287=CARTESIAN_POINT('Ctrl Pts',(-189.981745013892,89.4907965997159,-5.89197005329973));
#28288=CARTESIAN_POINT('Ctrl Pts',(-189.655066849744,89.9229556307455,-5.73799546302966));
#28289=CARTESIAN_POINT('Ctrl Pts',(-189.326983490681,90.3520514824435,-5.57410111969077));
#28290=CARTESIAN_POINT('Ctrl Pts',(-188.997857715772,90.7777088121816,-5.3973851824285));
#28291=CARTESIAN_POINT('Ctrl Pts',(-188.775987395932,91.0646529991488,-5.27825740663509));
#28292=CARTESIAN_POINT('Ctrl Pts',(-188.553790413721,91.3498385361321,-5.1533706364117));
#28293=CARTESIAN_POINT('Ctrl Pts',(-188.332426130858,91.6318520768341,-5.02200062463247));
#28294=CARTESIAN_POINT('Ctrl Pts',(-188.225415301687,91.7681816709206,-4.95849438185974));
#28295=CARTESIAN_POINT('Ctrl Pts',(-188.118599682122,91.9037704920273,-4.89347306955748));
#28296=CARTESIAN_POINT('Ctrl Pts',(-188.012113626743,92.0384616157055,-4.82685487001534));
#28297=CARTESIAN_POINT('Ctrl Pts',(-187.746746782362,92.3741164423341,-4.66084006809688));
#28298=CARTESIAN_POINT('Ctrl Pts',(-187.482921186823,92.7048308672381,-4.48476227846315));
#28299=CARTESIAN_POINT('Ctrl Pts',(-187.221786938517,93.029395239841,-4.29514604930913));
#28300=CARTESIAN_POINT('Ctrl Pts',(-187.16136829591,93.1044897131185,-4.25127453396387));
#28301=CARTESIAN_POINT('Ctrl Pts',(-187.101093892561,93.1792551071998,-4.20667827755538));
#28302=CARTESIAN_POINT('Ctrl Pts',(-187.040978266996,93.2536767007252,-4.16131423409769));
#28303=CARTESIAN_POINT('Ctrl Pts',(-186.822264168965,93.5244391114808,-3.99626969277047));
#28304=CARTESIAN_POINT('Ctrl Pts',(-186.60557949658,93.790733324454,-3.82129133643407));
#28305=CARTESIAN_POINT('Ctrl Pts',(-186.392328671109,94.0510234661448,-3.63203987613659));
#28306=CARTESIAN_POINT('Ctrl Pts',(-186.293631092486,94.1714919645312,-3.54444977729014));
#28307=CARTESIAN_POINT('Ctrl Pts',(-186.195669634349,94.2906748481443,-3.45380229447933));
#28308=CARTESIAN_POINT('Ctrl Pts',(-186.098586341438,94.4084223188913,-3.35966723216558));
#28309=CARTESIAN_POINT('Ctrl Pts',(-185.966190956342,94.5689980602577,-3.23129243715974));
#28310=CARTESIAN_POINT('Ctrl Pts',(-185.834880990427,94.7275622180069,-3.09597884224675));
#28311=CARTESIAN_POINT('Ctrl Pts',(-185.706791881215,94.8816114060829,-2.95260056874952));
#28312=CARTESIAN_POINT('Ctrl Pts',(-185.572843211037,95.042707724199,-2.8026633165852));
#28313=CARTESIAN_POINT('Ctrl Pts',(-185.442416968954,95.1988666121742,-2.64390665578969));
#28314=CARTESIAN_POINT('Ctrl Pts',(-185.317999081605,95.3472624190148,-2.4750430182964));
#28315=CARTESIAN_POINT('Ctrl Pts',(-185.285649188078,95.3858468111261,-2.43113678576129));
#28316=CARTESIAN_POINT('Ctrl Pts',(-185.25370570196,95.4239065608026,-2.38654726910167));
#28317=CARTESIAN_POINT('Ctrl Pts',(-185.22221274141,95.4613923628908,-2.3412518354128));
#28318=CARTESIAN_POINT('Ctrl Pts',(-185.100635614399,95.6061045792706,-2.16639089511405));
#28319=CARTESIAN_POINT('Ctrl Pts',(-184.98542456809,95.7426706963575,-1.98055943370035));
#28320=CARTESIAN_POINT('Ctrl Pts',(-184.880016161317,95.867230027294,-1.7782718643602));
#28321=CARTESIAN_POINT('Ctrl Pts',(-184.869055232791,95.8801823710909,-1.75723692362779));
#28322=CARTESIAN_POINT('Ctrl Pts',(-184.858200333914,95.8930049161292,-1.73602404382374));
#28323=CARTESIAN_POINT('Ctrl Pts',(-184.847455350633,95.905693340827,-1.71462705701883));
#28324=CARTESIAN_POINT('Ctrl Pts',(-184.733378649987,96.0404030549373,-1.48746079769588));
#28325=CARTESIAN_POINT('Ctrl Pts',(-184.634606015397,96.15654553355,-1.24506065412383));
#28326=CARTESIAN_POINT('Ctrl Pts',(-184.559925794379,96.2441998630232,-0.982882582956073));
#28327=CARTESIAN_POINT('Ctrl Pts',(-184.522585683869,96.2880270277597,-0.851793547372224));
#28328=CARTESIAN_POINT('Ctrl Pts',(-184.491200496658,96.3248129826987,-0.71446995864745));
#28329=CARTESIAN_POINT('Ctrl Pts',(-184.468141456029,96.3518258459007,-0.575828787863998));
#28330=CARTESIAN_POINT('Ctrl Pts',(-184.445082415399,96.3788387091026,-0.437187617080504));
#28331=CARTESIAN_POINT('Ctrl Pts',(-184.430008139983,96.3964802963479,-0.29639152936448));
#28332=CARTESIAN_POINT('Ctrl Pts',(-184.423682240228,96.4038839485828,-0.153238376079624));
#28333=CARTESIAN_POINT('Ctrl Pts',(-184.417356340473,96.4112876008179,-0.0100852227948052));
#28334=CARTESIAN_POINT('Ctrl Pts',(-184.42006841148,96.408114875489,0.135625753676425));
#28335=CARTESIAN_POINT('Ctrl Pts',(-184.43135369862,96.3949047695855,0.276911155354654));
#28336=CARTESIAN_POINT('Ctrl Pts',(-184.442638985761,96.3816946636821,0.418196557032899));
#28337=CARTESIAN_POINT('Ctrl Pts',(-184.462339979552,96.3586308331086,0.556826534586012));
#28338=CARTESIAN_POINT('Ctrl Pts',(-184.489631932353,96.3266448140663,0.69305600086679));
#28339=CARTESIAN_POINT('Ctrl Pts',(-184.516923885154,96.294658795024,0.829285467147568));
#28340=CARTESIAN_POINT('Ctrl Pts',(-184.552177704994,96.2533138975323,0.964043576315172));
#28341=CARTESIAN_POINT('Ctrl Pts',(-184.5930207893,96.2053417784222,1.09284689451645));
#28342=CARTESIAN_POINT('Ctrl Pts',(-184.633863873607,96.1573696593121,1.22165021271772));
#28343=CARTESIAN_POINT('Ctrl Pts',(-184.680332525911,96.1027279897818,1.3452763845494));
#28344=CARTESIAN_POINT('Ctrl Pts',(-184.731342004596,96.0426400031113,1.46469528137978));
#28345=CARTESIAN_POINT('Ctrl Pts',(-184.806244825786,95.9544062113289,1.64005116633558));
#28346=CARTESIAN_POINT('Ctrl Pts',(-184.890988249303,95.8543655363102,1.80625356976928));
#28347=CARTESIAN_POINT('Ctrl Pts',(-184.981448115991,95.7472408523625,1.96283299189215));
#28348=CARTESIAN_POINT('Ctrl Pts',(-185.014196175743,95.7084598362128,2.0195174914331));
#28349=CARTESIAN_POINT('Ctrl Pts',(-185.047693759096,95.6687507118301,2.07494083470269));
#28350=CARTESIAN_POINT('Ctrl Pts',(-185.081746563357,95.6283387304002,2.12908074636339));
#28351=CARTESIAN_POINT('Ctrl Pts',(-185.209863326123,95.476296854548,2.33277117271976));
#28352=CARTESIAN_POINT('Ctrl Pts',(-185.347035066172,95.3128818079577,2.52072565082259));
#28353=CARTESIAN_POINT('Ctrl Pts',(-185.490287760292,95.1413922088622,2.69775019367684));
#28354=CARTESIAN_POINT('Ctrl Pts',(-185.6117572313,94.9959795797082,2.84785611460146));
#28355=CARTESIAN_POINT('Ctrl Pts',(-185.738091612429,94.844170547157,2.99046782053365));
#28356=CARTESIAN_POINT('Ctrl Pts',(-185.866969235358,94.6886391437972,3.12595992617305));
#28357=CARTESIAN_POINT('Ctrl Pts',(-185.890080968629,94.6607475655074,3.15025784023058));
#28358=CARTESIAN_POINT('Ctrl Pts',(-185.913274594529,94.6327363650839,3.17432679112757));
#28359=CARTESIAN_POINT('Ctrl Pts',(-185.936536862367,94.6046210817755,3.19816893934182));
#28360=CARTESIAN_POINT('Ctrl Pts',(-186.132399677713,94.3678970193877,3.39891421085154));
#28361=CARTESIAN_POINT('Ctrl Pts',(-186.33318700497,94.1237178420589,3.58426602215573));
#28362=CARTESIAN_POINT('Ctrl Pts',(-186.537347521913,93.8737371558285,3.7581436355622));
#28363=CARTESIAN_POINT('Ctrl Pts',(-186.652107529757,93.7332213208283,3.85588141844489));
#28364=CARTESIAN_POINT('Ctrl Pts',(-186.767934004726,93.5908730084738,3.94999376768016));
#28365=CARTESIAN_POINT('Ctrl Pts',(-186.884556928866,93.4469907241288,4.04117676585312));
#28366=CARTESIAN_POINT('Ctrl Pts',(-187.102775149859,93.1777663297489,4.21179323592527));
#28367=CARTESIAN_POINT('Ctrl Pts',(-187.322831812982,92.9043391410468,4.37109190838243));
#28368=CARTESIAN_POINT('Ctrl Pts',(-187.543491073221,92.6281267656026,4.52125345487312));
#28369=CARTESIAN_POINT('Ctrl Pts',(-187.650554852589,92.4941086383265,4.5941117734665));
#28370=CARTESIAN_POINT('Ctrl Pts',(-187.757761085074,92.3594353231351,4.6648190424016));
#28371=CARTESIAN_POINT('Ctrl Pts',(-187.864972028382,92.2242715800883,4.73362434893738));
#28372=CARTESIAN_POINT('Ctrl Pts',(-188.193145537924,91.8105343388161,4.94423791341334));
#28373=CARTESIAN_POINT('Ctrl Pts',(-188.522111622863,91.3912547978073,5.13734380348656));
#28374=CARTESIAN_POINT('Ctrl Pts',(-188.850942384682,90.9673968784446,5.31766757924549));
#28375=CARTESIAN_POINT('Origin',(-192.01137155147,93.4192711577907,5.31766757925036));
#28376=CARTESIAN_POINT('Origin',(-192.27014422543,-93.0847597593693,-5.4533811546917));
#28377=CARTESIAN_POINT('Origin',(0.,-222.,0.));
#28378=CARTESIAN_POINT('',(199.738310248729,-222.,14.));
#28379=CARTESIAN_POINT('',(0.,-222.,14.));
#28380=CARTESIAN_POINT('Origin',(199.738310248729,-222.,0.));
#28381=CARTESIAN_POINT('Origin',(199.738310248729,222.,0.));
#28382=CARTESIAN_POINT('',(199.738310248729,222.,-14.));
#28383=CARTESIAN_POINT('Origin',(199.738310248729,222.,0.));
#28384=CARTESIAN_POINT('',(199.738310248729,222.,-14.));
#28385=CARTESIAN_POINT('Ctrl Pts',(-188.311118109849,-90.0308913574651,
-5.4533811546917));
#28386=CARTESIAN_POINT('Ctrl Pts',(-188.023256533701,-90.4040742676823,
-6.95129107926417));
#28387=CARTESIAN_POINT('Ctrl Pts',(-188.497959509479,-91.2585968975267,
-8.18023862635663));
#28388=CARTESIAN_POINT('Ctrl Pts',(-187.982864381004,-90.4564385369785,
-5.27854386264169));
#28389=CARTESIAN_POINT('Ctrl Pts',(-187.690945735358,-90.8320759397691,
-6.72011486605825));
#28390=CARTESIAN_POINT('Ctrl Pts',(-188.112012071841,-91.6642006348184,
-7.91797096057072));
#28391=CARTESIAN_POINT('Ctrl Pts',(-187.655409171816,-90.876129304024,-5.09218567437125));
#28392=CARTESIAN_POINT('Ctrl Pts',(-187.3584086985,-91.2554874222619,-6.4746919750007));
#28393=CARTESIAN_POINT('Ctrl Pts',(-187.72718172021,-92.0634779561488,-7.6384374977848));
#28394=CARTESIAN_POINT('Ctrl Pts',(-187.004381777406,-91.7014919148641,
-4.68919575393491));
#28395=CARTESIAN_POINT('Ctrl Pts',(-186.697275840756,-92.0880272032448,
-5.94749868714714));
#28396=CARTESIAN_POINT('Ctrl Pts',(-186.962365167593,-92.8473379257022,
-7.03394292888026));
#28397=CARTESIAN_POINT('Ctrl Pts',(-186.680764536156,-92.1072147831329,
-4.47270326949046));
#28398=CARTESIAN_POINT('Ctrl Pts',(-186.368574011069,-92.4973363451042,
-5.66609145238058));
#28399=CARTESIAN_POINT('Ctrl Pts',(-186.582338053018,-93.2319556715026,
-6.70919866065647));
#28400=CARTESIAN_POINT('Ctrl Pts',(-186.041188703775,-92.9007087164244,
-3.99710358616408));
#28401=CARTESIAN_POINT('Ctrl Pts',(-185.718995817204,-93.2976548774544,
-5.05164861453889));
#28402=CARTESIAN_POINT('Ctrl Pts',(-185.831571633446,-93.9828534973759,
-5.99578623488975));
#28403=CARTESIAN_POINT('Ctrl Pts',(-185.725094679122,-93.288633082395,-3.73845962749167));
#28404=CARTESIAN_POINT('Ctrl Pts',(-185.397870201454,-93.6890041414562,
-4.7194370719052));
#28405=CARTESIAN_POINT('Ctrl Pts',(-185.460673954076,-94.3492762075906,
-5.60781290938695));
#28406=CARTESIAN_POINT('Ctrl Pts',(-185.26239384512,-93.8509141779562,-3.29959059468005));
#28407=CARTESIAN_POINT('Ctrl Pts',(-184.927254687052,-94.2568244120627,
-4.15809811654345));
#28408=CARTESIAN_POINT('Ctrl Pts',(-184.917956107225,-94.8794830727165,
-4.94949632679128));
#28409=CARTESIAN_POINT('Ctrl Pts',(-185.110100842455,-94.0350359525012,
-3.14470232541573));
#28410=CARTESIAN_POINT('Ctrl Pts',(-184.772547238992,-94.4425242407308,
-3.96077463262501));
#28411=CARTESIAN_POINT('Ctrl Pts',(-184.739361183769,-95.0529459454586,
-4.7171591757551));
#28412=CARTESIAN_POINT('Ctrl Pts',(-184.811378660606,-94.3944781767998,
-2.81104162227018));
#28413=CARTESIAN_POINT('Ctrl Pts',(-184.469109421573,-94.8050009590216,
-3.53678993922348));
#28414=CARTESIAN_POINT('Ctrl Pts',(-184.389112179675,-95.3912948695953,
-4.21665767553714));
#28415=CARTESIAN_POINT('Ctrl Pts',(-184.665079428327,-94.5696290815887,
-2.63230461390646));
#28416=CARTESIAN_POINT('Ctrl Pts',(-184.320469107015,-94.9816612329742,
-3.31021936162184));
#28417=CARTESIAN_POINT('Ctrl Pts',(-184.217610983093,-95.5560191001983,
-3.94854645547927));
#28418=CARTESIAN_POINT('Ctrl Pts',(-184.388187849506,-94.8997059913566,
-2.2486720114352));
#28419=CARTESIAN_POINT('Ctrl Pts',(-184.039194420781,-95.3145079035315,
-2.82506962104317));
#28420=CARTESIAN_POINT('Ctrl Pts',(-183.893075603405,-95.866206695358,-3.37308506758693));
#28421=CARTESIAN_POINT('Ctrl Pts',(-184.255927894453,-95.0566151233063,
-2.04158414607042));
#28422=CARTESIAN_POINT('Ctrl Pts',(-183.904793548771,-95.4727832060237,
-2.56373454159151));
#28423=CARTESIAN_POINT('Ctrl Pts',(-183.738087091486,-96.0135328517609,
-3.06244641605404));
#28424=CARTESIAN_POINT('Ctrl Pts',(-184.018381326421,-95.337442413618,-1.59313909222305));
#28425=CARTESIAN_POINT('Ctrl Pts',(-183.663477755893,-95.7559537126499,
-1.99898838883818));
#28426=CARTESIAN_POINT('Ctrl Pts',(-183.459757334003,-96.277039469216,-2.38976375451145));
#28427=CARTESIAN_POINT('Ctrl Pts',(-183.913817195825,-95.4605163133078,
-1.35404044643148));
#28428=CARTESIAN_POINT('Ctrl Pts',(-183.557189126045,-95.8801261409614,
-1.69836151638071));
#28429=CARTESIAN_POINT('Ctrl Pts',(-183.337262264464,-96.3924294146135,
-2.03110764218774));
#28430=CARTESIAN_POINT('Ctrl Pts',(-183.790170269781,-95.6057447562368,
-0.961207376336125));
#28431=CARTESIAN_POINT('Ctrl Pts',(-183.431532892932,-96.0266119307892,
-1.20506005246625));
#28432=CARTESIAN_POINT('Ctrl Pts',(-183.192424146606,-96.5285376692198,
-1.44184452599264));
#28433=CARTESIAN_POINT('Ctrl Pts',(-183.754299774836,-95.6478116998946,
-0.822876876377623));
#28434=CARTESIAN_POINT('Ctrl Pts',(-183.395083934597,-96.0690372751092,
-1.03150468099448));
#28435=CARTESIAN_POINT('Ctrl Pts',(-183.150408545955,-96.5679516794309,
-1.23434398753411));
#28436=CARTESIAN_POINT('Ctrl Pts',(-183.69902716988,-95.7125878059592,-0.540441124336129));
#28437=CARTESIAN_POINT('Ctrl Pts',(-183.338932219072,-96.1343505158706,
-0.677342088342398));
#28438=CARTESIAN_POINT('Ctrl Pts',(-183.085668751854,-96.6286349566287,
-0.810680543872514));
#28439=CARTESIAN_POINT('Ctrl Pts',(-183.679493142585,-95.7354542735151,
-0.396620730396645));
#28440=CARTESIAN_POINT('Ctrl Pts',(-183.319081792273,-96.1574129706951,
-0.497048550961574));
#28441=CARTESIAN_POINT('Ctrl Pts',(-183.062789945167,-96.6500520617893,
-0.594944942795723));
#28442=CARTESIAN_POINT('Ctrl Pts',(-183.658485069448,-95.7600444241304,
-0.103191726056088));
#28443=CARTESIAN_POINT('Ctrl Pts',(-183.29773947503,-96.1822068475422,-0.129318689522527));
#28444=CARTESIAN_POINT('Ctrl Pts',(-183.03818476333,-96.6730832760899,-0.154791192776197));
#28445=CARTESIAN_POINT('Ctrl Pts',(-183.657281213906,-95.7614526744861,
0.0472614384620889));
#28446=CARTESIAN_POINT('Ctrl Pts',(-183.296516085829,-96.1836271975658,
0.0592303429672961));
#28447=CARTESIAN_POINT('Ctrl Pts',(-183.036774812679,-96.6744020956455,
0.0708938077874082));
#28448=CARTESIAN_POINT('Ctrl Pts',(-183.673584361532,-95.742371119294,0.340679262059982));
#28449=CARTESIAN_POINT('Ctrl Pts',(-183.313078626216,-96.1643875627615,
0.42693279541692));
#28450=CARTESIAN_POINT('Ctrl Pts',(-183.055869410689,-96.6565304997003,
0.511030789142554));
#28451=CARTESIAN_POINT('Ctrl Pts',(-183.690857386544,-95.722154582619,0.48526389943555));
#28452=CARTESIAN_POINT('Ctrl Pts',(-183.330631578546,-96.1439976105343,
0.608171774735233));
#28453=CARTESIAN_POINT('Ctrl Pts',(-183.076099939953,-96.6375959224396,
0.727912784662916));
#28454=CARTESIAN_POINT('Ctrl Pts',(-183.742255432096,-95.6619321066489,
0.770500979870421));
#28455=CARTESIAN_POINT('Ctrl Pts',(-183.382847157453,-96.0832758362534,
0.96580994111752));
#28456=CARTESIAN_POINT('Ctrl Pts',(-183.136301021943,-96.5811807995018,
1.15577832611497));
#28457=CARTESIAN_POINT('Ctrl Pts',(-183.776157527914,-95.6221850412214,
0.909351028967857));
#28458=CARTESIAN_POINT('Ctrl Pts',(-183.417296348802,-96.0431898175952,
1.1399943994718));
#28459=CARTESIAN_POINT('Ctrl Pts',(-183.176010556326,-96.543942355829,1.36405821104099));
#28460=CARTESIAN_POINT('Ctrl Pts',(-183.855733792922,-95.528750005071,1.17450600394942));
#28461=CARTESIAN_POINT('Ctrl Pts',(-183.498137619005,-95.9489789521239,
1.47279411141771));
#28462=CARTESIAN_POINT('Ctrl Pts',(-183.269223772346,-96.4563802390939,
1.76179982405154));
#28463=CARTESIAN_POINT('Ctrl Pts',(-183.901618838555,-95.4748146345266,
1.30195095812007));
#28464=CARTESIAN_POINT('Ctrl Pts',(-183.544760523303,-95.8945852221131,
1.63286614073801));
#28465=CARTESIAN_POINT('Ctrl Pts',(-183.322974451362,-96.4058247503125,
1.9529716304919));
#28466=CARTESIAN_POINT('Ctrl Pts',(-184.003311269862,-95.3550653583824,
1.54843340014721));
#28467=CARTESIAN_POINT('Ctrl Pts',(-183.648068240509,-95.7738395791422,
1.94266932112714));
#28468=CARTESIAN_POINT('Ctrl Pts',(-183.442107513798,-96.2935423316836,
2.32270370778772));
#28469=CARTESIAN_POINT('Ctrl Pts',(-184.059298282184,-95.2890376172853,
1.66765797594319));
#28470=CARTESIAN_POINT('Ctrl Pts',(-183.704951723409,-95.7072529344379,
2.09265259025143));
#28471=CARTESIAN_POINT('Ctrl Pts',(-183.507700412238,-96.2316144996131,
2.50154461511258));
#28472=CARTESIAN_POINT('Ctrl Pts',(-184.176852645184,-95.1501214463336,
1.89427491600449));
#28473=CARTESIAN_POINT('Ctrl Pts',(-183.824371480539,-95.5671780822467,
2.37798322300348));
#28474=CARTESIAN_POINT('Ctrl Pts',(-183.645434899623,-96.1012760045966,
2.84147765793412));
#28475=CARTESIAN_POINT('Ctrl Pts',(-184.238711432394,-95.0768906699632,
2.00242188310459));
#28476=CARTESIAN_POINT('Ctrl Pts',(-183.887217279107,-95.4933286417111,
2.51428318649114));
#28477=CARTESIAN_POINT('Ctrl Pts',(-183.717917865943,-96.0325444858201,
3.00370172415377));
#28478=CARTESIAN_POINT('Ctrl Pts',(-184.431540341704,-94.8481206782299,
2.31455411749311));
#28479=CARTESIAN_POINT('Ctrl Pts',(-184.083210281331,-95.2625185890143,
2.90827578108584));
#28480=CARTESIAN_POINT('Ctrl Pts',(-183.943883949142,-95.8177457977801,
3.47191039252339));
#28481=CARTESIAN_POINT('Ctrl Pts',(-184.569662566592,-94.6836182645234,
2.50639205885069));
#28482=CARTESIAN_POINT('Ctrl Pts',(-184.223558056762,-95.096589316792,3.15082824084193));
#28483=CARTESIAN_POINT('Ctrl Pts',(-184.10576675548,-95.6631811146341,3.75967355830051));
#28484=CARTESIAN_POINT('Ctrl Pts',(-184.858717524764,-94.3376512020014,
2.86757408695932));
#28485=CARTESIAN_POINT('Ctrl Pts',(-184.517183278251,-94.7477114570037,
3.60852645239219));
#28486=CARTESIAN_POINT('Ctrl Pts',(-184.444611440482,-95.3378252413274,
4.30145816243324));
#28487=CARTESIAN_POINT('Ctrl Pts',(-185.008454788704,-94.1576148308574,
3.03519751519597));
#28488=CARTESIAN_POINT('Ctrl Pts',(-184.669304580449,-94.5661300912731,
3.8214674405414));
#28489=CARTESIAN_POINT('Ctrl Pts',(-184.620171995052,-95.168376829891,4.55289856427253));
#28490=CARTESIAN_POINT('Ctrl Pts',(-185.463984272662,-93.6071208020851,
3.50623173809894));
#28491=CARTESIAN_POINT('Ctrl Pts',(-185.132626075302,-94.010243710356,4.42215777302216));
#28492=CARTESIAN_POINT('Ctrl Pts',(-185.154364647646,-94.6497916478071,
5.25946424297357));
#28493=CARTESIAN_POINT('Ctrl Pts',(-185.777957045331,-93.2240351821244,
3.78096556311151));
#28494=CARTESIAN_POINT('Ctrl Pts',(-185.451626884343,-93.6237620559661,
4.77394349177421));
#28495=CARTESIAN_POINT('Ctrl Pts',(-185.522692219371,-94.2883029853266,
5.67157304213761));
#28496=CARTESIAN_POINT('Ctrl Pts',(-186.415826334264,-92.4372580682707,
4.28435082010938));
#28497=CARTESIAN_POINT('Ctrl Pts',(-186.099491131265,-92.8302396868848,
5.4221694834975));
#28498=CARTESIAN_POINT('Ctrl Pts',(-186.271292454703,-93.5444970023476,
6.42666499108573));
#28499=CARTESIAN_POINT('Ctrl Pts',(-186.739930459906,-92.033330946282,4.51235264699637));
#28500=CARTESIAN_POINT('Ctrl Pts',(-186.428710026573,-92.4227379511592,
5.71753872292767));
#28501=CARTESIAN_POINT('Ctrl Pts',(-186.651807929004,-93.161960330059,6.76867375764101));
#28502=CARTESIAN_POINT('Ctrl Pts',(-187.393530947007,-91.2095920430833,
4.9357741836659));
#28503=CARTESIAN_POINT('Ctrl Pts',(-187.092477352195,-91.5918564120394,
6.26953035299208));
#28504=CARTESIAN_POINT('Ctrl Pts',(-187.419481988969,-92.3803984155784,
7.40381660388869));
#28505=CARTESIAN_POINT('Ctrl Pts',(-187.723431876917,-90.789245324442,5.13113846604913));
#28506=CARTESIAN_POINT('Ctrl Pts',(-187.427506580947,-91.1677963691818,
6.52589394947526));
#28507=CARTESIAN_POINT('Ctrl Pts',(-187.807116502426,-91.9808618362968,
7.69686757472972));
#28508=CARTESIAN_POINT('Ctrl Pts',(-188.379735239133,-89.9434589515106,
5.49397424411016));
#28509=CARTESIAN_POINT('Ctrl Pts',(-188.093936031686,-90.3146004408659,
7.00530187354627));
#28510=CARTESIAN_POINT('Ctrl Pts',(-188.578584928303,-91.1754925110962,
8.24112908982782));
#28511=CARTESIAN_POINT('Ctrl Pts',(-188.707031074314,-89.5169094143503,
5.66196658593984));
#28512=CARTESIAN_POINT('Ctrl Pts',(-188.426255795464,-89.8842722210176,
7.22884474588428));
#28513=CARTESIAN_POINT('Ctrl Pts',(-188.963467607895,-90.7686092384922,
8.49312094838692));
#28514=CARTESIAN_POINT('Ctrl Pts',(-189.68511297814,-88.2275681149711,6.13501898387808));
#28515=CARTESIAN_POINT('Ctrl Pts',(-189.422317700218,-88.5795741093693,
7.86491570906493));
#28516=CARTESIAN_POINT('Ctrl Pts',(-190.114092759895,-89.5365583941309,
9.20270785472519));
#28517=CARTESIAN_POINT('Ctrl Pts',(-190.332033957746,-87.3551470887722,
6.40961295144101));
#28518=CARTESIAN_POINT('Ctrl Pts',(-190.078977721377,-87.6992096958193,
8.23877620276131));
#28519=CARTESIAN_POINT('Ctrl Pts',(-190.875743827135,-88.7000469473906,
9.61460278261497));
#28520=CARTESIAN_POINT('Ctrl Pts',(-191.611898320755,-85.5882580977726,
6.90461427888993));
#28521=CARTESIAN_POINT('Ctrl Pts',(-191.378062267531,-85.9164296154525,
8.92407374163879));
#28522=CARTESIAN_POINT('Ctrl Pts',(-192.383730616602,-87.0002198715461,
10.3571100610023));
#28523=CARTESIAN_POINT('Ctrl Pts',(-192.244891171766,-84.693736712425,7.12463735632059));
#28524=CARTESIAN_POINT('Ctrl Pts',(-192.020340574275,-85.0137142395017,
9.23418963052937));
#28525=CARTESIAN_POINT('Ctrl Pts',(-193.130124103834,-86.1368550460551,
10.6871461172942));
#28526=CARTESIAN_POINT('Ctrl Pts',(-194.119961067917,-81.9797996678922,
7.72418030763564));
#28527=CARTESIAN_POINT('Ctrl Pts',(-193.934940664567,-82.257849756744,10.1010557721888));
#28528=CARTESIAN_POINT('Ctrl Pts',(-195.342719172301,-83.50920211737,11.5864611755336));
#28529=CARTESIAN_POINT('Ctrl Pts',(-195.338006413608,-80.1301500968197,
8.04415647990219));
#28530=CARTESIAN_POINT('Ctrl Pts',(-195.16935199361,-80.3905659076323,10.5812896754235));
#28531=CARTESIAN_POINT('Ctrl Pts',(-196.782194293857,-81.7074776699032,
12.0664230083597));
#28532=CARTESIAN_POINT('Ctrl Pts',(-197.110239250038,-77.3006000230673,
8.44922123457134));
#28533=CARTESIAN_POINT('Ctrl Pts',(-196.954831995167,-77.5532375792707,
11.2157823096582));
#28534=CARTESIAN_POINT('Ctrl Pts',(-198.879361941047,-78.935681607343,12.6740132502263));
#28535=CARTESIAN_POINT('Ctrl Pts',(-197.692624677484,-76.3469248856778,
8.5715135010636));
#28536=CARTESIAN_POINT('Ctrl Pts',(-197.544944403591,-76.5909251985067,
11.414061030348));
#28537=CARTESIAN_POINT('Ctrl Pts',(-199.569000827311,-77.9989242812487,
12.8574486612482));
#28538=CARTESIAN_POINT('Ctrl Pts',(-198.833501317186,-74.43002371175,8.79383680878653));
#28539=CARTESIAN_POINT('Ctrl Pts',(-198.701046000336,-74.6567602970987,
11.7854080990333));
#28540=CARTESIAN_POINT('Ctrl Pts',(-200.920841970448,-76.1111237379196,
13.1909267424754));
#28541=CARTESIAN_POINT('Ctrl Pts',(-199.392274367538,-73.4664233641185,
8.89394683892845));
#28542=CARTESIAN_POINT('Ctrl Pts',(-199.266893542384,-73.6846080389232,
11.9582237199827));
#28543=CARTESIAN_POINT('Ctrl Pts',(-201.583376310003,-75.1597219207058,
13.3410879530753));
#28544=CARTESIAN_POINT('Ctrl Pts',(-201.033783983709,-70.5604287764574,
9.16677201385106));
#28545=CARTESIAN_POINT('Ctrl Pts',(-200.940109283218,-70.7339672756153,
12.4488343143003));
#28546=CARTESIAN_POINT('Ctrl Pts',(-203.530870313903,-72.2835771071226,
13.7503128604518));
#28547=CARTESIAN_POINT('Ctrl Pts',(-202.081723044656,-68.6028539641832,
9.31223534268044));
#28548=CARTESIAN_POINT('Ctrl Pts',(-201.999085118096,-68.7598621453509,
12.7310897529191));
#28549=CARTESIAN_POINT('Ctrl Pts',(-204.775735293809,-70.3369061379169,
13.9684983839894));
#28550=CARTESIAN_POINT('Ctrl Pts',(-204.085562846173,-64.6481906295588,
9.55122215804647));
#28551=CARTESIAN_POINT('Ctrl Pts',(-204.026314097882,-64.7713562775311,
13.238108357264));
#28552=CARTESIAN_POINT('Ctrl Pts',(-207.158618873108,-66.387628113296,14.3269579904162));
#28553=CARTESIAN_POINT('Ctrl Pts',(-205.041466127102,-62.6510984859536,
9.64459843558729));
#28554=CARTESIAN_POINT('Ctrl Pts',(-204.990809880274,-62.7587308992531,
13.4607910313532));
#28555=CARTESIAN_POINT('Ctrl Pts',(-208.296641479989,-64.3850167536084,
14.4670115183672));
#28556=CARTESIAN_POINT('Ctrl Pts',(-207.771662686836,-56.601430798315,9.86749344214829));
#28557=CARTESIAN_POINT('Ctrl Pts',(-207.783522326383,-56.5847268119357,
14.0716577550469));
#28558=CARTESIAN_POINT('Ctrl Pts',(-211.550002283707,-58.2963858291117,
14.8013197394809));
#28559=CARTESIAN_POINT('Ctrl Pts',(-209.408693149567,-52.4905952748467,
9.94066884240314));
#28560=CARTESIAN_POINT('Ctrl Pts',(-209.420079879466,-52.454626832127,14.3810813496773));
#28561=CARTESIAN_POINT('Ctrl Pts',(-213.504906168685,-54.1297053236517,
14.9110597099366));
#28562=CARTESIAN_POINT('Ctrl Pts',(-212.31378134909,-44.1146587717776,10.0094381670403));
#28563=CARTESIAN_POINT('Ctrl Pts',(-212.345419819919,-44.0267219078386,
14.9024839573744));
#28564=CARTESIAN_POINT('Ctrl Pts',(-216.978639285811,-45.5934511118201,
15.0141686414793));
#28565=CARTESIAN_POINT('Ctrl Pts',(-213.581879775254,-39.8495543519757,
10.0043954519828));
#28566=CARTESIAN_POINT('Ctrl Pts',(-213.605139445775,-39.7586824716392,
15.1062312896536));
#28567=CARTESIAN_POINT('Ctrl Pts',(-218.497528523746,-41.2238500697657,
15.0065832746786));
#28568=CARTESIAN_POINT('Ctrl Pts',(-214.929428919574,-34.4198302895606,
9.97920576186122));
#28569=CARTESIAN_POINT('Ctrl Pts',(-214.936859859468,-34.3891593318107,
15.3153703026194));
#28570=CARTESIAN_POINT('Ctrl Pts',(-220.113030275332,-35.6397174849627,
14.9687749372571));
#28571=CARTESIAN_POINT('Ctrl Pts',(-215.187043011382,-33.3287590530146,
9.97318130845427));
#28572=CARTESIAN_POINT('Ctrl Pts',(-215.19468682512,-33.2957346146807,15.3553818376476));
#28573=CARTESIAN_POINT('Ctrl Pts',(-220.421957075912,-34.5165678200411,
14.9597336598784));
#28574=CARTESIAN_POINT('Ctrl Pts',(-215.675983586131,-31.1472549362169,
9.95985565385693));
#28575=CARTESIAN_POINT('Ctrl Pts',(-215.68418616737,-31.1095679945434,15.4307038587473));
#28576=CARTESIAN_POINT('Ctrl Pts',(-221.008423709188,-32.2690261896159,
14.9397363624086));
#28577=CARTESIAN_POINT('Ctrl Pts',(-215.90764622814,-30.055516718288,9.95254907226967));
#28578=CARTESIAN_POINT('Ctrl Pts',(-215.915775634413,-30.0163642711029,
15.4659963578014));
#28579=CARTESIAN_POINT('Ctrl Pts',(-221.286366523007,-31.1432926323065,
14.9287722668472));
#28580=CARTESIAN_POINT('Ctrl Pts',(-216.564558495436,-26.7773677629292,
9.92956539341713));
#28581=CARTESIAN_POINT('Ctrl Pts',(-216.575423316015,-26.7202845042959,
15.5658559264057));
#28582=CARTESIAN_POINT('Ctrl Pts',(-222.074674899071,-27.7605386096942,
14.8942846816766));
#28583=CARTESIAN_POINT('Ctrl Pts',(-216.951752658587,-24.5880241878653,
9.91285560896527));
#28584=CARTESIAN_POINT('Ctrl Pts',(-216.960777488742,-24.5333219085994,
15.6232654891544));
#28585=CARTESIAN_POINT('Ctrl Pts',(-222.539542982626,-25.4979652324832,
14.8692127365989));
#28586=CARTESIAN_POINT('Ctrl Pts',(-217.963118570905,-18.0083995826229,
9.86431151401665));
#28587=CARTESIAN_POINT('Ctrl Pts',(-217.976908530276,-17.9105064968268,
15.7736929532904));
#28588=CARTESIAN_POINT('Ctrl Pts',(-223.754139848201,-18.6905621049579,
14.7963774439254));
#28589=CARTESIAN_POINT('Ctrl Pts',(-218.43737553185,-13.6065465446901,9.83453026560912));
#28590=CARTESIAN_POINT('Ctrl Pts',(-218.441702505744,-13.5485089098786,
15.8411776329903));
#28591=CARTESIAN_POINT('Ctrl Pts',(-224.324191182824,-14.1260707926592,
14.7516962153847));
#28592=CARTESIAN_POINT('Ctrl Pts',(-218.989193202051,-4.7721628047025,9.79912404537101));
#28593=CARTESIAN_POINT('Ctrl Pts',(-218.990897585228,-4.7335129665023,15.9210896224386));
#28594=CARTESIAN_POINT('Ctrl Pts',(-224.987517064859,-4.95696670963562,
14.6985760232229));
#28595=CARTESIAN_POINT('Ctrl Pts',(-219.066759730313,-0.339632492972661,
9.79351850252103));
#28596=CARTESIAN_POINT('Ctrl Pts',(-219.066727564461,-0.350430413971326,
15.9320679979825));
#28597=CARTESIAN_POINT('Ctrl Pts',(-225.080801055053,-0.352320764338334,
14.6901661447284));
#28598=CARTESIAN_POINT('Ctrl Pts',(-218.880718901755,6.33255501405285,9.8059454221472));
#28599=CARTESIAN_POINT('Ctrl Pts',(-218.881432931089,6.31289977575216,15.9051486662368));
#28600=CARTESIAN_POINT('Ctrl Pts',(-224.857132572439,6.57614298146129,14.7088102047727));
#28601=CARTESIAN_POINT('Ctrl Pts',(-218.768230359849,8.56052172271425,9.81343805284001));
#28602=CARTESIAN_POINT('Ctrl Pts',(-218.770003081734,8.53077447021609,15.8889618235594));
#28603=CARTESIAN_POINT('Ctrl Pts',(-224.721894016949,8.88921878827596,14.7200513807027));
#28604=CARTESIAN_POINT('Ctrl Pts',(-218.522448524829,11.9084288001204,9.82890166451567));
#28605=CARTESIAN_POINT('Ctrl Pts',(-218.524928042834,11.8774402237096,15.8532704560566));
#28606=CARTESIAN_POINT('Ctrl Pts',(-224.426467103965,12.3631418548612,14.7432516194942));
#28607=CARTESIAN_POINT('Ctrl Pts',(-218.427625255158,13.0254701659967,9.83475451805377));
#28608=CARTESIAN_POINT('Ctrl Pts',(-218.430609970526,12.991870685901,15.8395230780581));
#28609=CARTESIAN_POINT('Ctrl Pts',(-224.312498386649,13.5219155099691,14.7520327570961));
#28610=CARTESIAN_POINT('Ctrl Pts',(-218.21323860133,15.2503993161315,9.84754794127491));
#28611=CARTESIAN_POINT('Ctrl Pts',(-218.217068753284,15.2132620015528,15.8083419032611));
#28612=CARTESIAN_POINT('Ctrl Pts',(-224.054856092527,15.8291500128444,14.7712270705584));
#28613=CARTESIAN_POINT('Ctrl Pts',(-218.093583727244,16.3596870431594,9.85449428714121));
#28614=CARTESIAN_POINT('Ctrl Pts',(-218.097966645082,16.3205496369381,15.7909263232461));
#28615=CARTESIAN_POINT('Ctrl Pts',(-223.911072517391,16.979063905479,14.7816489139371));
#28616=CARTESIAN_POINT('Ctrl Pts',(-217.433606562207,21.8903944208552,9.89118647408106));
#28617=CARTESIAN_POINT('Ctrl Pts',(-217.445236527621,21.8024400591546,15.6952267122392));
#28618=CARTESIAN_POINT('Ctrl Pts',(-223.118121902026,22.7098222865059,14.8366999810007));
#28619=CARTESIAN_POINT('Ctrl Pts',(-216.708563916788,26.2647200848804,9.92732876816586));
#28620=CARTESIAN_POINT('Ctrl Pts',(-216.731935048167,26.1494884159972,15.5904394521733));
#28621=CARTESIAN_POINT('Ctrl Pts',(-222.247281590068,27.2343164729745,14.8909272767638));
#28622=CARTESIAN_POINT('Ctrl Pts',(-214.873442978039,34.9151616307584,9.98467680865938));
#28623=CARTESIAN_POINT('Ctrl Pts',(-214.895229142084,34.8173622853258,15.310263695862));
#28624=CARTESIAN_POINT('Ctrl Pts',(-220.045590647228,36.1539662505485,14.9769827670247));
#28625=CARTESIAN_POINT('Ctrl Pts',(-213.763346868112,39.1912731419991,10.0059888635648));
#28626=CARTESIAN_POINT('Ctrl Pts',(-213.795786303056,39.0868620241777,15.1393495471316));
#28627=CARTESIAN_POINT('Ctrl Pts',(-218.71471064539,40.5491477077801,15.0089703691583));
#28628=CARTESIAN_POINT('Ctrl Pts',(-211.157664540089,47.6451012812898,9.99106655001459));
#28629=CARTESIAN_POINT('Ctrl Pts',(-211.176219821159,47.5841008473432,14.6986672737439));
#28630=CARTESIAN_POINT('Ctrl Pts',(-215.595563893305,49.1983243309679,14.9866296990289));
#28631=CARTESIAN_POINT('Ctrl Pts',(-209.662098742207,51.8228239014422,9.95531537582467));
#28632=CARTESIAN_POINT('Ctrl Pts',(-209.685532101084,51.7729467688604,14.4360702739088));
#28633=CARTESIAN_POINT('Ctrl Pts',(-213.80730640242,53.4523572352619,14.9330257980933));
#28634=CARTESIAN_POINT('Ctrl Pts',(-207.545508834274,56.9818337014807,9.83445365866236));
#28635=CARTESIAN_POINT('Ctrl Pts',(-207.510723871588,57.0648634396861,14.0005580141263));
#28636=CARTESIAN_POINT('Ctrl Pts',(-211.281520603173,58.6720114070539,14.7517626507157));
#28637=CARTESIAN_POINT('Ctrl Pts',(-207.109809764703,58.0104721219209,9.80639282881937));
#28638=CARTESIAN_POINT('Ctrl Pts',(-207.071261697803,58.1008397078743,13.9102924731027));
#28639=CARTESIAN_POINT('Ctrl Pts',(-210.761813438706,59.7110402643347,14.7096772084586));
#28640=CARTESIAN_POINT('Ctrl Pts',(-206.213392812189,60.0613541485855,9.74108338571072));
#28641=CARTESIAN_POINT('Ctrl Pts',(-206.166184591471,60.1672120878568,13.7184889746833));
#28642=CARTESIAN_POINT('Ctrl Pts',(-209.693081442639,61.7790036523918,14.6117245857318));
#28643=CARTESIAN_POINT('Ctrl Pts',(-205.752839497752,61.08313643902,9.70383665509273));
#28644=CARTESIAN_POINT('Ctrl Pts',(-205.701230510568,61.1968025962474,13.6171538768307));
#28645=CARTESIAN_POINT('Ctrl Pts',(-209.144253544922,62.8074679437847,14.5558602053489));
#28646=CARTESIAN_POINT('Ctrl Pts',(-204.339722003525,64.1253772453607,9.57651965325937));
#28647=CARTESIAN_POINT('Ctrl Pts',(-204.282123111009,64.2443553233843,13.2971569314029));
#28648=CARTESIAN_POINT('Ctrl Pts',(-207.461156573031,65.8638453333561,14.3649014156848));
#28649=CARTESIAN_POINT('Ctrl Pts',(-203.353817729955,66.1271301231815,9.47090861847069));
#28650=CARTESIAN_POINT('Ctrl Pts',(-203.286815403105,66.2623803486336,13.0595360566483));
#28651=CARTESIAN_POINT('Ctrl Pts',(-206.288029158072,67.867179527562,14.2064955657256));
#28652=CARTESIAN_POINT('Ctrl Pts',(-201.295982075669,70.0773663077491,9.20351075942536));
#28653=CARTESIAN_POINT('Ctrl Pts',(-201.204273063212,70.2469450403615,12.51897904355));
#28654=CARTESIAN_POINT('Ctrl Pts',(-203.84229300212,71.8036809549284,13.8054187109848));
#28655=CARTESIAN_POINT('Ctrl Pts',(-200.224040052249,72.0258588331287,9.04188770997817));
#28656=CARTESIAN_POINT('Ctrl Pts',(-200.12047497987,72.2124872803002,12.2182147537059));
#28657=CARTESIAN_POINT('Ctrl Pts',(-202.569671040505,73.7368570614262,13.5629930900514));
#28658=CARTESIAN_POINT('Ctrl Pts',(-197.995685176027,75.8684360666186,8.64078280222561));
#28659=CARTESIAN_POINT('Ctrl Pts',(-197.862702838989,76.0899116945249,11.5260954437677));
#28660=CARTESIAN_POINT('Ctrl Pts',(-199.927578782646,77.5306853270276,12.9613510241432));
#28661=CARTESIAN_POINT('Ctrl Pts',(-196.839245861665,77.7625466240603,8.40173977014487));
#28662=CARTESIAN_POINT('Ctrl Pts',(-196.691996019402,78.0013102762491,11.1379598928392));
#28663=CARTESIAN_POINT('Ctrl Pts',(-198.558076797564,79.3913614209033,12.60279242272));
#28664=CARTESIAN_POINT('Ctrl Pts',(-195.042731573518,80.5611850737664,7.95715194188054));
#28665=CARTESIAN_POINT('Ctrl Pts',(-194.858551738376,80.8435039704777,10.4503583874007));
#28666=CARTESIAN_POINT('Ctrl Pts',(-196.433609218416,82.125363186609,11.9359168266832));
#28667=CARTESIAN_POINT('Ctrl Pts',(-194.433589268338,81.4869661634149,7.79447520514001));
#28668=CARTESIAN_POINT('Ctrl Pts',(-194.240902692785,81.7777231153474,10.2062460954892));
#28669=CARTESIAN_POINT('Ctrl Pts',(-195.713756493118,83.0271859261819,11.6919029300314));
#28670=CARTESIAN_POINT('Ctrl Pts',(-193.195101021216,83.3238217818029,7.43221244759254));
#28671=CARTESIAN_POINT('Ctrl Pts',(-192.984483082209,83.6312855291968,9.67471802243613));
#28672=CARTESIAN_POINT('Ctrl Pts',(-194.251251280249,84.8111598877124,11.1485096657566));
#28673=CARTESIAN_POINT('Ctrl Pts',(-192.565602902613,84.2350179279496,7.23258583606902));
#28674=CARTESIAN_POINT('Ctrl Pts',(-192.345875521816,84.5508501176059,9.38782701439113));
#28675=CARTESIAN_POINT('Ctrl Pts',(-193.508421789667,85.6934162800533,10.8490693154141));
#28676=CARTESIAN_POINT('Ctrl Pts',(-191.295766122429,86.0299410528198,6.78753527123933));
#28677=CARTESIAN_POINT('Ctrl Pts',(-191.057182564862,86.3619994488762,8.76050448431005));
#28678=CARTESIAN_POINT('Ctrl Pts',(-192.011112251812,87.4258398244962,10.1814905385105));
#28679=CARTESIAN_POINT('Ctrl Pts',(-190.654477805639,86.9150843481393,6.54205946398291));
#28680=CARTESIAN_POINT('Ctrl Pts',(-190.406326530197,87.25527815843,8.42065139010884));
#28681=CARTESIAN_POINT('Ctrl Pts',(-191.255510732542,88.2773832319173,9.81327421990134));
#28682=CARTESIAN_POINT('Ctrl Pts',(-189.349584768406,88.6752321827888,5.98095856523893));
#28683=CARTESIAN_POINT('Ctrl Pts',(-189.081798171609,89.0309342903906,7.65676092118989));
#28684=CARTESIAN_POINT('Ctrl Pts',(-189.719216239347,89.9651010967815,8.97161470628148));
#28685=CARTESIAN_POINT('Ctrl Pts',(-188.685650085394,89.5498148663974,5.66466085148541));
#28686=CARTESIAN_POINT('Ctrl Pts',(-188.407635601515,89.9135939257602,7.23283181006476));
#28687=CARTESIAN_POINT('Ctrl Pts',(-188.93805424261,90.8008600150856,8.49708749073966));
#28688=CARTESIAN_POINT('Ctrl Pts',(-188.020722526437,90.4061090473696,5.2954583188303));
#28689=CARTESIAN_POINT('Ctrl Pts',(-187.728390752002,90.7825752206079,6.74229702851374));
#28690=CARTESIAN_POINT('Ctrl Pts',(-188.15658149337,91.6160251236586,7.94335562892809));
#28691=CARTESIAN_POINT('',(-188.06083509298,90.3544283086146,5.31766757924143));
#28692=CARTESIAN_POINT('',(-188.311118109849,-90.0308913574651,-5.4533811546917));
#28693=CARTESIAN_POINT('Ctrl Pts',(-188.06083509298,90.3544283086146,5.31766757924145));
#28694=CARTESIAN_POINT('Ctrl Pts',(-188.51680197023,89.7666938435659,5.56940638867454));
#28695=CARTESIAN_POINT('Ctrl Pts',(-188.972498711518,89.1700935523622,5.79657748555383));
#28696=CARTESIAN_POINT('Ctrl Pts',(-189.426627535133,88.5659108843427,6.00556125304925));
#28697=CARTESIAN_POINT('Ctrl Pts',(-189.619911580624,88.3087616698077,6.09450788211784));
#28698=CARTESIAN_POINT('Ctrl Pts',(-189.81291152598,88.050239085108,6.18016056957736));
#28699=CARTESIAN_POINT('Ctrl Pts',(-190.00552702852,87.7904427618453,6.26301392151901));
#28700=CARTESIAN_POINT('Ctrl Pts',(-190.0065706244,87.7890351785042,6.26346282316814));
#28701=CARTESIAN_POINT('Ctrl Pts',(-190.007614208963,87.7876275578147,6.26391164261233));
#28702=CARTESIAN_POINT('Ctrl Pts',(-190.008657782195,87.7862198997925,6.26436037993047));
#28703=CARTESIAN_POINT('Ctrl Pts',(-190.573087725994,87.0248700354609,6.50706570388179));
#28704=CARTESIAN_POINT('Ctrl Pts',(-191.13430700821,86.2524813601324,6.72525538225101));
#28705=CARTESIAN_POINT('Ctrl Pts',(-191.691014022882,85.4702469629432,6.9250607165503));
#28706=CARTESIAN_POINT('Ctrl Pts',(-191.769609740418,85.359811361975,6.95326916947602));
#28707=CARTESIAN_POINT('Ctrl Pts',(-191.848115518518,85.249179541194,6.98111127249217));
#28708=CARTESIAN_POINT('Ctrl Pts',(-191.926527692939,85.1383548791639,7.00860435543439));
#28709=CARTESIAN_POINT('Ctrl Pts',(-191.92791329294,85.1363965269951,7.00909017815311));
#28710=CARTESIAN_POINT('Ctrl Pts',(-191.929298863927,85.1344381143097,7.00957589192428));
#28711=CARTESIAN_POINT('Ctrl Pts',(-191.930684405876,85.1324796411284,7.01006149684292));
#28712=CARTESIAN_POINT('Ctrl Pts',(-192.487088704112,84.3459982959562,7.20507014607013));
#28713=CARTESIAN_POINT('Ctrl Pts',(-193.039539566412,83.5486706128072,7.3825606229965));
#28714=CARTESIAN_POINT('Ctrl Pts',(-193.584625019812,82.7450778439038,7.5454311084043));
#28715=CARTESIAN_POINT('Ctrl Pts',(-193.660087593468,82.6338270700391,7.56797918031646));
#28716=CARTESIAN_POINT('Ctrl Pts',(-193.735409008233,82.5224562631648,7.59024711098675));
#28717=CARTESIAN_POINT('Ctrl Pts',(-193.810580221864,82.4109776165522,7.61224265150016));
#28718=CARTESIAN_POINT('Ctrl Pts',(-193.81183523018,82.4091164436146,7.61260987433606));
#28719=CARTESIAN_POINT('Ctrl Pts',(-193.813090196661,82.4072552405714,7.61297702124396));
#28720=CARTESIAN_POINT('Ctrl Pts',(-193.814345121268,82.4053940074768,7.6133440922604));
#28721=CARTESIAN_POINT('Ctrl Pts',(-194.432553090273,81.4885029645941,7.79417266663633));
#28722=CARTESIAN_POINT('Ctrl Pts',(-195.040750453091,80.5641977261954,7.95662373930324));
#28723=CARTESIAN_POINT('Ctrl Pts',(-195.638717557925,79.6327484802435,8.10464224532399));
#28724=CARTESIAN_POINT('Ctrl Pts',(-195.639668281456,79.6312675447386,8.10487758381603));
#28725=CARTESIAN_POINT('Ctrl Pts',(-195.640618979127,79.6297865911748,8.10511288582298));
#28726=CARTESIAN_POINT('Ctrl Pts',(-195.641569650937,79.6283056195534,8.1053481513607));
#28727=CARTESIAN_POINT('Ctrl Pts',(-196.838915668809,77.763061004687,8.40165887801138));
#28728=CARTESIAN_POINT('Ctrl Pts',(-197.99521745823,75.8692128806453,8.64068943479255));
#28729=CARTESIAN_POINT('Ctrl Pts',(-199.109366290497,73.9480033042068,8.84124604920835));
#28730=CARTESIAN_POINT('Ctrl Pts',(-199.109531730703,73.947718023373,8.84127582990427));
#28731=CARTESIAN_POINT('Ctrl Pts',(-199.109697169979,73.9474327419359,8.84130560975191));
#28732=CARTESIAN_POINT('Ctrl Pts',(-199.109862608326,73.9471474598955,8.84133538875136));
#28733=CARTESIAN_POINT('Ctrl Pts',(-200.223942142281,72.026027669517,9.04187035788895));
#28734=CARTESIAN_POINT('Ctrl Pts',(-201.29590104568,70.0775218531977,9.20350054478848));
#28735=CARTESIAN_POINT('Ctrl Pts',(-202.324899898542,68.1022482236617,9.33720984811441));
#28736=CARTESIAN_POINT('Ctrl Pts',(-202.325616587401,68.1008724625512,9.33730297549529));
#28737=CARTESIAN_POINT('Ctrl Pts',(-202.326333255426,68.0994966884513,9.33739608925299));
#28738=CARTESIAN_POINT('Ctrl Pts',(-202.327049902617,68.0981209013622,9.33748918939001));
#28739=CARTESIAN_POINT('Ctrl Pts',(-203.355125526122,66.1244674934296,9.47104721167366));
#28740=CARTESIAN_POINT('Ctrl Pts',(-204.340330517151,64.1240672021237,9.57657447788188));
#28741=CARTESIAN_POINT('Ctrl Pts',(-205.28180033275,62.0972167083591,9.66139767126757));
#28742=CARTESIAN_POINT('Ctrl Pts',(-205.283387201231,62.0938004064126,9.66154064266165));
#28743=CARTESIAN_POINT('Ctrl Pts',(-205.284973950805,62.0903840168381,9.66168355513634));
#28744=CARTESIAN_POINT('Ctrl Pts',(-205.286560581401,62.0869675397905,9.66182640871456));
#28745=CARTESIAN_POINT('Ctrl Pts',(-205.755928257212,61.0762824471217,9.70408630975619));
#28746=CARTESIAN_POINT('Ctrl Pts',(-206.214896939989,60.0579129054442,9.74119304854463));
#28747=CARTESIAN_POINT('Ctrl Pts',(-206.661601287996,59.0359131362846,9.77373814714519));
#28748=CARTESIAN_POINT('Ctrl Pts',(-206.663590354042,59.031362419351,9.77388306257059));
#28749=CARTESIAN_POINT('Ctrl Pts',(-206.66557917369,59.0268116395308,9.7740278875185));
#28750=CARTESIAN_POINT('Ctrl Pts',(-206.667567746947,59.0222607968317,9.77417262205041));
#28751=CARTESIAN_POINT('Ctrl Pts',(-207.113676431887,58.0013426866808,9.8066417963464));
#28752=CARTESIAN_POINT('Ctrl Pts',(-207.547387284822,56.9772551360114,9.83456186917772));
#28753=CARTESIAN_POINT('Ctrl Pts',(-207.968826809702,55.9500317564852,9.85862677614977));
#28754=CARTESIAN_POINT('Ctrl Pts',(-207.971163590813,55.9443360491565,9.85876021028857));
#28755=CARTESIAN_POINT('Ctrl Pts',(-207.973499995396,55.9386402456129,9.85889352833538));
#28756=CARTESIAN_POINT('Ctrl Pts',(-207.975836023462,55.9329443458578,9.85902673037562));
#28757=CARTESIAN_POINT('Ctrl Pts',(-209.666224089052,51.8112982462088,9.95541390241721));
#28758=CARTESIAN_POINT('Ctrl Pts',(-211.159461284655,47.6392719557561,9.99108029052597));
#28759=CARTESIAN_POINT('Ctrl Pts',(-212.460505703252,43.4181872143984,9.99852947308981));
#28760=CARTESIAN_POINT('Ctrl Pts',(-212.463715926966,43.4077720232338,9.99854785335583));
#28761=CARTESIAN_POINT('Ctrl Pts',(-212.466924980455,43.3973565333573,9.99856605889622));
#28762=CARTESIAN_POINT('Ctrl Pts',(-212.470132863722,43.3869407447705,9.99858409003113));
#28763=CARTESIAN_POINT('Ctrl Pts',(-213.768815578448,39.1702023323294,10.0058838329716));
#28764=CARTESIAN_POINT('Ctrl Pts',(-214.875703511897,34.9045058683299,9.9846099748668));
#28765=CARTESIAN_POINT('Ctrl Pts',(-215.791003449954,30.589940845844,9.95600474013346));
#28766=CARTESIAN_POINT('Ctrl Pts',(-215.794260322957,30.5745885118635,9.95590295533826));
#28767=CARTESIAN_POINT('Ctrl Pts',(-215.797514770452,30.559235559204,9.95580107637761));
#28768=CARTESIAN_POINT('Ctrl Pts',(-215.800766792235,30.5438819878149,9.95569910388854));
#28769=CARTESIAN_POINT('Ctrl Pts',(-216.713708471003,26.2336663211255,9.92707231675218));
#28770=CARTESIAN_POINT('Ctrl Pts',(-217.435480651459,21.8746892726661,9.8910825901607));
#28771=CARTESIAN_POINT('Ctrl Pts',(-217.961588294286,17.4658285182826,9.86183279026221));
#28772=CARTESIAN_POINT('Ctrl Pts',(-217.964035693427,17.445318947339,9.86169672317379));
#28773=CARTESIAN_POINT('Ctrl Pts',(-217.966478850021,17.4248082947604,9.86156079087027));
#28774=CARTESIAN_POINT('Ctrl Pts',(-217.968917763295,17.4042965603517,9.86142499435562));
#28775=CARTESIAN_POINT('Ctrl Pts',(-218.098016566448,16.318550547643,9.85423688820197));
#28776=CARTESIAN_POINT('Ctrl Pts',(-218.215230776192,15.2297242981946,9.84742921466242));
#28777=CARTESIAN_POINT('Ctrl Pts',(-218.320431928289,14.1379347405934,9.84115131508478));
#28778=CARTESIAN_POINT('Ctrl Pts',(-218.322535801835,14.1161005009297,9.84102576601444));
#28779=CARTESIAN_POINT('Ctrl Pts',(-218.324634906511,14.0942645369404,9.84090042657939));
#28780=CARTESIAN_POINT('Ctrl Pts',(-218.326729238281,14.0724268925217,9.84077529794832));
#28781=CARTESIAN_POINT('Ctrl Pts',(-218.431337469398,12.981674516305,9.83452534034928));
#28782=CARTESIAN_POINT('Ctrl Pts',(-218.524056391673,11.8865273086927,9.82880091068774));
#28783=CARTESIAN_POINT('Ctrl Pts',(-218.604375803264,10.7924597730254,9.82374741828564));
#28784=CARTESIAN_POINT('Ctrl Pts',(-218.606072766715,10.7693446557215,9.82364064967597));
#28785=CARTESIAN_POINT('Ctrl Pts',(-218.60776421916,10.7462299863214,9.82353418301963));
#28786=CARTESIAN_POINT('Ctrl Pts',(-218.609450161518,10.7231157661814,9.82342801890493));
#28787=CARTESIAN_POINT('Ctrl Pts',(-218.770554963031,8.51437367592111,9.81328321855358));
#28788=CARTESIAN_POINT('Ctrl Pts',(-218.881361170861,6.30952061087333,9.80590609607315));
#28789=CARTESIAN_POINT('Ctrl Pts',(-218.942732511399,4.10849250724635,9.80180559598378));
#28790=CARTESIAN_POINT('Ctrl Pts',(-218.94344205954,4.08304519935568,9.80175818782569));
#28791=CARTESIAN_POINT('Ctrl Pts',(-218.94414500976,4.05759840202034,9.80171123365064));
#28792=CARTESIAN_POINT('Ctrl Pts',(-218.944841362669,4.03215211519381,9.80166473310975));
#28793=CARTESIAN_POINT('Ctrl Pts',(-219.065865799387,-0.390350456036404,
9.79358305254647));
#28794=CARTESIAN_POINT('Ctrl Pts',(-218.987614587639,-4.79743579236434,
9.7992336121286));
#28795=CARTESIAN_POINT('Ctrl Pts',(-218.713284367982,-9.18935465820405,
9.81683142676904));
#28796=CARTESIAN_POINT('Ctrl Pts',(-218.711406729688,-9.21941490843551,
9.81695187405592));
#28797=CARTESIAN_POINT('Ctrl Pts',(-218.709519905522,-9.24947444815586,
9.81707288013222));
#28798=CARTESIAN_POINT('Ctrl Pts',(-218.70762389497,-9.27953327733394,9.81719444199773));
#28799=CARTESIAN_POINT('Ctrl Pts',(-218.430911254125,-13.666459284364,9.8349357487566));
#28800=CARTESIAN_POINT('Ctrl Pts',(-217.95852998986,-18.0382514286823,9.86453422912174));
#28801=CARTESIAN_POINT('Ctrl Pts',(-217.288874630294,-22.3948159800386,
9.89667511604252));
#28802=CARTESIAN_POINT('Ctrl Pts',(-217.283555754183,-22.4294188944924,
9.89693040168043));
#28803=CARTESIAN_POINT('Ctrl Pts',(-217.278224413937,-22.4640208469283,
9.89718581860337));
#28804=CARTESIAN_POINT('Ctrl Pts',(-217.272880606905,-22.4986218371657,
9.89744135928248));
#28805=CARTESIAN_POINT('Ctrl Pts',(-216.939522261105,-24.6571071266348,
9.91338254457614));
#28806=CARTESIAN_POINT('Ctrl Pts',(-216.557648993695,-26.8118478251854,
9.92980747149138));
#28807=CARTESIAN_POINT('Ctrl Pts',(-216.126616984069,-28.9628003990182,
9.94488797127757));
#28808=CARTESIAN_POINT('Ctrl Pts',(-216.119233106746,-28.9996477086767,
9.94514631069991));
#28809=CARTESIAN_POINT('Ctrl Pts',(-216.111834797523,-29.0364939062531,
9.94540424670578));
#28810=CARTESIAN_POINT('Ctrl Pts',(-216.104422051958,-29.0733389914415,
9.9456617682015));
#28811=CARTESIAN_POINT('Ctrl Pts',(-215.892008213258,-30.1291429326299,
9.95304110275137));
#28812=CARTESIAN_POINT('Ctrl Pts',(-215.667723636287,-31.1841083198772,
9.96008078617996));
#28813=CARTESIAN_POINT('Ctrl Pts',(-215.431513298767,-32.2380069945684,
9.96651848957129));
#28814=CARTESIAN_POINT('Ctrl Pts',(-215.423005023906,-32.2759683289206,
9.96675037506158));
#28815=CARTESIAN_POINT('Ctrl Pts',(-215.414480871154,-32.3139298605291,
9.96698148614846));
#28816=CARTESIAN_POINT('Ctrl Pts',(-215.40594089593,-32.3518913495086,9.96721180811115));
#28817=CARTESIAN_POINT('Ctrl Pts',(-215.16911597409,-33.4046141530769,9.97359894383225));
#28818=CARTESIAN_POINT('Ctrl Pts',(-214.920050029317,-34.457620960072,9.97938362263439));
#28819=CARTESIAN_POINT('Ctrl Pts',(-214.659919093045,-35.5057750926369,
9.98424592547359));
#28820=CARTESIAN_POINT('Ctrl Pts',(-214.650247074172,-35.5447468762224,
9.98442671244765));
#28821=CARTESIAN_POINT('Ctrl Pts',(-214.64055978287,-35.5837122211703,9.9846062788195));
#28822=CARTESIAN_POINT('Ctrl Pts',(-214.630857226511,-35.622671116418,9.98478460672069));
#28823=CARTESIAN_POINT('Ctrl Pts',(-213.559099608934,-39.9261238571264,
10.0044829500703));
#28824=CARTESIAN_POINT('Ctrl Pts',(-212.300728554187,-44.1522925375462,
10.0091555454261));
#28825=CARTESIAN_POINT('Ctrl Pts',(-210.861237215767,-48.302627120132,9.97506716298549));
#28826=CARTESIAN_POINT('Ctrl Pts',(-210.846648861139,-48.3446881948322,
9.97472169830747));
#28827=CARTESIAN_POINT('Ctrl Pts',(-210.832041900486,-48.386741481317,9.97437231709957));
#28828=CARTESIAN_POINT('Ctrl Pts',(-210.817416335251,-48.4287869789396,
9.97401898219888));
#28829=CARTESIAN_POINT('Ctrl Pts',(-209.375759165835,-52.5732553885937,
9.93919039372426));
#28830=CARTESIAN_POINT('Ctrl Pts',(-207.753330793897,-56.642051284793,9.86601251598906));
#28831=CARTESIAN_POINT('Ctrl Pts',(-205.951531538682,-60.6345428301356,
9.71890487965252));
#28832=CARTESIAN_POINT('Ctrl Pts',(-205.931370267354,-60.6792168997281,
9.71725881560739));
#28833=CARTESIAN_POINT('Ctrl Pts',(-205.91118650737,-60.7238813995598,9.71560338632713));
#28834=CARTESIAN_POINT('Ctrl Pts',(-205.890980256884,-60.7685363263265,
9.71393851524477));
#28835=CARTESIAN_POINT('Ctrl Pts',(-204.999073030556,-62.7396121526445,
9.64045083130972));
#28836=CARTESIAN_POINT('Ctrl Pts',(-204.063345493926,-64.6920375334682,
9.54857804243365));
#28837=CARTESIAN_POINT('Ctrl Pts',(-203.083642786703,-66.6255226101039,
9.43173548532964));
#28838=CARTESIAN_POINT('Ctrl Pts',(-202.081695627481,-68.6029080614775,
9.31223998194527));
#28839=CARTESIAN_POINT('Ctrl Pts',(-201.033751116317,-70.5604869697111,
9.16677491688292));
#28840=CARTESIAN_POINT('Ctrl Pts',(-199.939444119453,-72.4977587142569,
8.98489165361757));
#28841=CARTESIAN_POINT('Ctrl Pts',(-199.91309919235,-72.5443976218348,8.98051289946019));
#28842=CARTESIAN_POINT('Ctrl Pts',(-199.88672738753,-72.5910247522546,8.97611289164215));
#28843=CARTESIAN_POINT('Ctrl Pts',(-199.860328698315,-72.6376400958351,
8.97169142002573));
#28844=CARTESIAN_POINT('Ctrl Pts',(-199.338431354915,-73.5592170642366,
8.88427972046174));
#28845=CARTESIAN_POINT('Ctrl Pts',(-198.806014126144,-74.4762076967677,
8.78848127769314));
#28846=CARTESIAN_POINT('Ctrl Pts',(-198.263062970022,-75.3884743446064,
8.68267570895607));
#28847=CARTESIAN_POINT('Ctrl Pts',(-198.235092082578,-75.4354710356309,
8.67722498724615));
#28848=CARTESIAN_POINT('Ctrl Pts',(-198.207092562445,-75.4824560900013,
8.67174751883111));
#28849=CARTESIAN_POINT('Ctrl Pts',(-198.179064838505,-75.5294288251994,
8.66624311624193));
#28850=CARTESIAN_POINT('Ctrl Pts',(-197.635470254205,-76.4404597928872,
8.55948584106465));
#28851=CARTESIAN_POINT('Ctrl Pts',(-197.08120557516,-77.3469552823971,8.44262055412659));
#28852=CARTESIAN_POINT('Ctrl Pts',(-196.519493300536,-78.2437860485531,
8.31422647338811));
#28853=CARTESIAN_POINT('Ctrl Pts',(-196.490056260816,-78.2907852758758,
8.30749786547763));
#28854=CARTESIAN_POINT('Ctrl Pts',(-196.460596833056,-78.3377612230074,
8.30073821556141));
#28855=CARTESIAN_POINT('Ctrl Pts',(-196.431115108733,-78.3847138039004,
8.29394705947406));
#28856=CARTESIAN_POINT('Ctrl Pts',(-195.695048802598,-79.5569726718873,
8.1243931649728));
#28857=CARTESIAN_POINT('Ctrl Pts',(-194.945007563397,-80.7147865676449,
7.9352916044913));
#28858=CARTESIAN_POINT('Ctrl Pts',(-194.182159059277,-81.8572132916295,
7.71947409973443));
#28859=CARTESIAN_POINT('Ctrl Pts',(-193.748804736262,-82.5061960934465,
7.59687380863673));
#28860=CARTESIAN_POINT('Ctrl Pts',(-193.311317539902,-83.1502134702393,
7.46565285377205));
#28861=CARTESIAN_POINT('Ctrl Pts',(-192.869912506659,-83.7890938733829,
7.32450466033796));
#28862=CARTESIAN_POINT('Ctrl Pts',(-192.838362656537,-83.8347584658703,
7.31441595719134));
#28863=CARTESIAN_POINT('Ctrl Pts',(-192.80679286958,-83.8803967263716,7.304275914378));
#28864=CARTESIAN_POINT('Ctrl Pts',(-192.775203283695,-83.9260085284507,
7.29408359580739));
#28865=CARTESIAN_POINT('Ctrl Pts',(-192.266915439948,-84.6599188941247,
7.13008550960481));
#28866=CARTESIAN_POINT('Ctrl Pts',(-191.753495353972,-85.3869876622751,
6.95261874682967));
#28867=CARTESIAN_POINT('Ctrl Pts',(-191.235538330077,-86.1066609025267,
6.75770746303479));
#28868=CARTESIAN_POINT('Ctrl Pts',(-191.147808666634,-86.2285565198139,
6.72469410374118));
#28869=CARTESIAN_POINT('Ctrl Pts',(-191.059948858487,-86.3502399712669,
6.69118041028271));
#28870=CARTESIAN_POINT('Ctrl Pts',(-190.971961813689,-86.4717085650345,
6.65714721763566));
#28871=CARTESIAN_POINT('Ctrl Pts',(-190.939875691232,-86.5160043608901,
6.64473637704678));
#28872=CARTESIAN_POINT('Ctrl Pts',(-190.90777252411,-86.560271718568,6.63225741831689));
#28873=CARTESIAN_POINT('Ctrl Pts',(-190.875652557489,-86.6045103960844,
6.61970860958682));
#28874=CARTESIAN_POINT('Ctrl Pts',(-190.401447417493,-87.2576308838022,
6.43444348553252));
#28875=CARTESIAN_POINT('Ctrl Pts',(-189.923571498165,-87.9045121020593,
6.23403435388213));
#28876=CARTESIAN_POINT('Ctrl Pts',(-189.442826746467,-88.5443600219234,
6.01293258678423));
#28877=CARTESIAN_POINT('Ctrl Pts',(-189.306461275911,-88.725855841416,5.95021604873683));
#28878=CARTESIAN_POINT('Ctrl Pts',(-189.169864992924,-88.9067857888991,
5.88583489329034));
#28879=CARTESIAN_POINT('Ctrl Pts',(-189.033056229673,-89.0871318100725,
5.8196632777581));
#28880=CARTESIAN_POINT('Ctrl Pts',(-189.001009116442,-89.1293774179127,
5.80416274105795));
#28881=CARTESIAN_POINT('Ctrl Pts',(-188.96895048776,-89.1715908315416,5.78856285244983));
#28882=CARTESIAN_POINT('Ctrl Pts',(-188.936880751009,-89.2137716331804,
5.77286066138358));
#28883=CARTESIAN_POINT('Ctrl Pts',(-188.683433073572,-89.547127229166,5.64876597712418));
#28884=CARTESIAN_POINT('Ctrl Pts',(-188.429224761621,-89.8785325446022,
5.51826779476947));
#28885=CARTESIAN_POINT('Ctrl Pts',(-188.174626035996,-90.2075623578002,
5.37998727999571));
#28886=CARTESIAN_POINT('Ctrl Pts',(-188.133621029437,-90.2605550411505,
5.35771618102844));
#28887=CARTESIAN_POINT('Ctrl Pts',(-188.092605902664,-90.313486129659,5.33524331946663));
#28888=CARTESIAN_POINT('Ctrl Pts',(-188.05158220932,-90.3663538760784,5.31256306641583));
#28889=CARTESIAN_POINT('Ctrl Pts',(-188.019880255481,-90.4072085802729,
5.29503640617024));
#28890=CARTESIAN_POINT('Ctrl Pts',(-187.988164848065,-90.4480358164431,
5.27738103636211));
#28891=CARTESIAN_POINT('Ctrl Pts',(-187.956440707941,-90.4888298148183,
5.259595025775));
#28892=CARTESIAN_POINT('Ctrl Pts',(-187.75306131691,-90.7503549031177,5.14557119446294));
#28893=CARTESIAN_POINT('Ctrl Pts',(-187.549103864686,-91.0107947425876,
5.02608364485494));
#28894=CARTESIAN_POINT('Ctrl Pts',(-187.345892263011,-91.268521005334,4.90062671379455));
#28895=CARTESIAN_POINT('Ctrl Pts',(-187.25263651765,-91.386794049459,4.84305332959621));
#28896=CARTESIAN_POINT('Ctrl Pts',(-187.159537867347,-91.5044957625111,
4.78422344319158));
#28897=CARTESIAN_POINT('Ctrl Pts',(-187.066723847658,-91.6214701352587,
4.72409173688634));
#28898=CARTESIAN_POINT('Ctrl Pts',(-187.035938485457,-91.6602692137318,
4.70414672895975));
#28899=CARTESIAN_POINT('Ctrl Pts',(-187.005180842154,-91.6989930300589,
4.68405900940515));
#28900=CARTESIAN_POINT('Ctrl Pts',(-186.974453572332,-91.7376387068004,
4.66382280836529));
#28901=CARTESIAN_POINT('Ctrl Pts',(-186.781298812858,-91.9805693817015,
4.53661597979979));
#28902=CARTESIAN_POINT('Ctrl Pts',(-186.589254838546,-92.2205246511467,
4.40358022722448));
#28903=CARTESIAN_POINT('Ctrl Pts',(-186.398878611342,-92.4569161279226,
4.26313874687862));
#28904=CARTESIAN_POINT('Ctrl Pts',(-186.297709583587,-92.582538408742,4.18850585688057));
#28905=CARTESIAN_POINT('Ctrl Pts',(-186.197011499421,-92.7071543463695,
4.11178235875304));
#28906=CARTESIAN_POINT('Ctrl Pts',(-186.096867627569,-92.8306763058842,
4.03273768018468));
#28907=CARTESIAN_POINT('Ctrl Pts',(-186.068151779818,-92.8660957251426,
4.01007194025181));
#28908=CARTESIAN_POINT('Ctrl Pts',(-186.039479816593,-92.9014271072812,
3.98722064024348));
#28909=CARTESIAN_POINT('Ctrl Pts',(-186.010855777804,-92.9366660656645,
3.96417195795104));
#28910=CARTESIAN_POINT('Ctrl Pts',(-185.865981518665,-93.1150202813691,
3.84751613604557));
#28911=CARTESIAN_POINT('Ctrl Pts',(-185.722265707347,-93.2910917770091,
3.72582451668043));
#28912=CARTESIAN_POINT('Ctrl Pts',(-185.580307265502,-93.4642190437351,
3.59764267842825));
#28913=CARTESIAN_POINT('Ctrl Pts',(-185.450978642463,-93.6219434504375,
3.48086497627492));
#28914=CARTESIAN_POINT('Ctrl Pts',(-185.323108761286,-93.7772240998859,
3.35870017216342));
#28915=CARTESIAN_POINT('Ctrl Pts',(-185.197140819223,-93.9295753497621,
3.23009067295042));
#28916=CARTESIAN_POINT('Ctrl Pts',(-185.184839193751,-93.944453484512,3.21753108147375));
#28917=CARTESIAN_POINT('Ctrl Pts',(-185.172555697486,-93.9593036951516,
3.20491006625581));
#28918=CARTESIAN_POINT('Ctrl Pts',(-185.160290736874,-93.9741255382158,
3.19222666815781));
#28919=CARTESIAN_POINT('Ctrl Pts',(-185.135032506227,-94.0046493647953,
3.16610671517324));
#28920=CARTESIAN_POINT('Ctrl Pts',(-185.109840003889,-94.0350683943748,
3.13970033206727));
#28921=CARTESIAN_POINT('Ctrl Pts',(-185.084727989822,-94.0653655712933,
3.11299775843998));
#28922=CARTESIAN_POINT('Ctrl Pts',(-185.000757625597,-94.1666742506354,
3.02370882975576));
#28923=CARTESIAN_POINT('Ctrl Pts',(-184.917546304095,-94.2667902418731,
2.93098623593855));
#28924=CARTESIAN_POINT('Ctrl Pts',(-184.835738044685,-94.3649633720747,
2.83451960455793));
#28925=CARTESIAN_POINT('Ctrl Pts',(-184.794841327897,-94.4140410413836,
2.78629503002805));
#28926=CARTESIAN_POINT('Ctrl Pts',(-184.754295103115,-94.4626333930311,
2.73713544658652));
#28927=CARTESIAN_POINT('Ctrl Pts',(-184.714178396369,-94.5106486763438,
2.68700652086778));
#28928=CARTESIAN_POINT('Ctrl Pts',(-184.691560089061,-94.5377203011496,
2.65874319770587));
#28929=CARTESIAN_POINT('Ctrl Pts',(-184.669107579012,-94.5645735297545,
2.63021393443707));
#28930=CARTESIAN_POINT('Ctrl Pts',(-184.646834983318,-94.5911925894902,
2.60140281589878));
#28931=CARTESIAN_POINT('Ctrl Pts',(-184.558200755562,-94.697123655435,2.48674840931461));
#28932=CARTESIAN_POINT('Ctrl Pts',(-184.472336938954,-94.7994405101602,
2.36757759974578));
#28933=CARTESIAN_POINT('Ctrl Pts',(-184.39001361699,-94.8972907412225,2.24276030558802));
#28934=CARTESIAN_POINT('Ctrl Pts',(-184.360538666391,-94.9323249290794,
2.19807086046513));
#28935=CARTESIAN_POINT('Ctrl Pts',(-184.331517390034,-94.966786755673,2.15265794738168));
#28936=CARTESIAN_POINT('Ctrl Pts',(-184.302984457013,-95.0006378956154,
2.10647100277846));
#28937=CARTESIAN_POINT('Ctrl Pts',(-184.284616631745,-95.0224292699243,
2.07673856246047));
#28938=CARTESIAN_POINT('Ctrl Pts',(-184.266453222769,-95.0439652433064,
2.04668207816586));
#28939=CARTESIAN_POINT('Ctrl Pts',(-184.248509638701,-95.0652285217695,
2.01627815072083));
#28940=CARTESIAN_POINT('Ctrl Pts',(-184.203571054875,-95.1184810725424,
1.94013341637187));
#28941=CARTESIAN_POINT('Ctrl Pts',(-184.160013235404,-95.1700208923274,
1.86181972998249));
#28942=CARTESIAN_POINT('Ctrl Pts',(-184.11807248382,-95.2195830531759,1.78097027598704));
#28943=CARTESIAN_POINT('Ctrl Pts',(-184.065729691486,-95.2814374977177,
1.68006874177653));
#28944=CARTESIAN_POINT('Ctrl Pts',(-184.015676542522,-95.3404806834878,
1.57462166859957));
#28945=CARTESIAN_POINT('Ctrl Pts',(-183.969546039874,-95.3948223314433,
1.46600813692336));
#28946=CARTESIAN_POINT('Ctrl Pts',(-183.963788790444,-95.4016043607678,
1.45245278509672));
#28947=CARTESIAN_POINT('Ctrl Pts',(-183.958092599144,-95.4083132066439,
1.43884808896023));
#28948=CARTESIAN_POINT('Ctrl Pts',(-183.952460605122,-95.4149452355462,
1.42519670863897));
#28949=CARTESIAN_POINT('Ctrl Pts',(-183.939870672291,-95.4297706771367,
1.39467999277968));
#28950=CARTESIAN_POINT('Ctrl Pts',(-183.92759053512,-95.4442253572866,1.36391850743349));
#28951=CARTESIAN_POINT('Ctrl Pts',(-183.91563674564,-95.4582906918077,1.33289908442677));
#28952=CARTESIAN_POINT('Ctrl Pts',(-183.888000177376,-95.4908090474554,
1.26118371727321));
#28953=CARTESIAN_POINT('Ctrl Pts',(-183.862086334608,-95.521271749357,1.18803365022812));
#28954=CARTESIAN_POINT('Ctrl Pts',(-183.838139395079,-95.5494024579498,
1.11341655287846));
#28955=CARTESIAN_POINT('Ctrl Pts',(-183.830539615712,-95.5583299945345,
1.08973613742647));
#28956=CARTESIAN_POINT('Ctrl Pts',(-183.823137717431,-95.5670229192437,
1.06590814401409));
#28957=CARTESIAN_POINT('Ctrl Pts',(-183.815940854834,-95.5754731656678,
1.04193206334385));
#28958=CARTESIAN_POINT('Ctrl Pts',(-183.807052112064,-95.5859099449995,
1.01231954666276));
#28959=CARTESIAN_POINT('Ctrl Pts',(-183.798465657636,-95.5959888299654,
0.982424266488826));
#28960=CARTESIAN_POINT('Ctrl Pts',(-183.790207377758,-95.6056800572553,
0.952284262991848));
#28961=CARTESIAN_POINT('Ctrl Pts',(-183.770637055188,-95.6286461527345,
0.880859026811543));
#28962=CARTESIAN_POINT('Ctrl Pts',(-183.752834291628,-95.6495237102342,
0.807724319669422));
#28963=CARTESIAN_POINT('Ctrl Pts',(-183.737174261358,-95.667880389908,0.733396237962366));
#28964=CARTESIAN_POINT('Ctrl Pts',(-183.729815806035,-95.6765059675685,
0.698470387944005));
#28965=CARTESIAN_POINT('Ctrl Pts',(-183.722930052581,-95.6845754234538,
0.663281346768663));
#28966=CARTESIAN_POINT('Ctrl Pts',(-183.716553371217,-95.6920469043472,
0.627883782731233));
#28967=CARTESIAN_POINT('Ctrl Pts',(-183.711527814294,-95.6979352889768,
0.599986438821077));
#28968=CARTESIAN_POINT('Ctrl Pts',(-183.706826946361,-95.7034423959074,
0.57202855141883));
#28969=CARTESIAN_POINT('Ctrl Pts',(-183.702455562656,-95.7085628613754,
0.544016869547344));
#28970=CARTESIAN_POINT('Ctrl Pts',(-183.690432620339,-95.7226460590806,
0.466974253730033));
#28971=CARTESIAN_POINT('Ctrl Pts',(-183.680879377209,-95.7338310775459,
0.389326927627816));
#28972=CARTESIAN_POINT('Ctrl Pts',(-183.673906168774,-95.7419938810966,
0.311176583107222));
#28973=CARTESIAN_POINT('Ctrl Pts',(-183.670430979897,-95.7460619201294,
0.272229345192594));
#28974=CARTESIAN_POINT('Ctrl Pts',(-183.667596074987,-95.7493799400455,
0.233157230799864));
#28975=CARTESIAN_POINT('Ctrl Pts',(-183.665411948407,-95.7519362878294,
0.193973187426416));
#28976=CARTESIAN_POINT('Ctrl Pts',(-183.664060507716,-95.7535180424976,
0.169727838683484));
#28977=CARTESIAN_POINT('Ctrl Pts',(-183.662964569235,-95.7548007725713,
0.145395417202572));
#28978=CARTESIAN_POINT('Ctrl Pts',(-183.662122791516,-95.7557860370457,
0.121013577556789));
#28979=CARTESIAN_POINT('Ctrl Pts',(-183.659349263018,-95.7590323323995,
0.0406791548507267));
#28980=CARTESIAN_POINT('Ctrl Pts',(-183.659369903306,-95.7590083849867,
-0.0405743786132426));
#28981=CARTESIAN_POINT('Ctrl Pts',(-183.662167137276,-95.7557343635116,
-0.121409031646972));
#28982=CARTESIAN_POINT('Ctrl Pts',(-183.66365575411,-95.7539920124849,-0.164427179750673));
#28983=CARTESIAN_POINT('Ctrl Pts',(-183.665930163209,-95.7513298702821,
-0.20732660630546));
#28984=CARTESIAN_POINT('Ctrl Pts',(-183.668983873669,-95.7477554733448,
-0.249907146204909));
#28985=CARTESIAN_POINT('Ctrl Pts',(-183.67039589183,-95.7461026927514,-0.269596143044668));
#28986=CARTESIAN_POINT('Ctrl Pts',(-183.671969627319,-95.7442605895704,
-0.289232202416622));
#28987=CARTESIAN_POINT('Ctrl Pts',(-183.673702142494,-95.7422325155245,
-0.308814502605387));
#28988=CARTESIAN_POINT('Ctrl Pts',(-183.683157232174,-95.7311644323959,
-0.415683641223018));
#28989=CARTESIAN_POINT('Ctrl Pts',(-183.697388129984,-95.7145027257029,
-0.521069269126041));
#28990=CARTESIAN_POINT('Ctrl Pts',(-183.716065692174,-95.6926183979358,
-0.625191032757183));
#28991=CARTESIAN_POINT('Ctrl Pts',(-183.719449769401,-95.6886533057849,
-0.64405624041201));
#28992=CARTESIAN_POINT('Ctrl Pts',(-183.722979909019,-95.6845166626267,
-0.66287994147631));
#28993=CARTESIAN_POINT('Ctrl Pts',(-183.726654266742,-95.680210541379,-0.681663421242707));
#28994=CARTESIAN_POINT('Ctrl Pts',(-183.729553586093,-95.6768127174321,
-0.696484870450501));
#28995=CARTESIAN_POINT('Ctrl Pts',(-183.732544154011,-95.6733076374794,
-0.711278140450021));
#28996=CARTESIAN_POINT('Ctrl Pts',(-183.735622809827,-95.6696989480456,
-0.726038309658969));
#28997=CARTESIAN_POINT('Ctrl Pts',(-183.754762108044,-95.6472645522066,
-0.817798901629893));
#28998=CARTESIAN_POINT('Ctrl Pts',(-183.777288708933,-95.6208459470195,
-0.908128526296283));
#28999=CARTESIAN_POINT('Ctrl Pts',(-183.802436490926,-95.5913270514141,
-0.995898950364328));
#29000=CARTESIAN_POINT('Ctrl Pts',(-183.811736072317,-95.5804110440969,
-1.02835621448973));
#29001=CARTESIAN_POINT('Ctrl Pts',(-183.821394374083,-95.5690707476792,
-1.06046321037403));
#29002=CARTESIAN_POINT('Ctrl Pts',(-183.831373372734,-95.5573500029804,
-1.09216144311939));
#29003=CARTESIAN_POINT('Ctrl Pts',(-183.834612567923,-95.5535454348907,
-1.10245072830553));
#29004=CARTESIAN_POINT('Ctrl Pts',(-183.837886716341,-95.5496994128863,
-1.11270736160523));
#29005=CARTESIAN_POINT('Ctrl Pts',(-183.84119544588,-95.5458123496254,-1.12293200011363));
#29006=CARTESIAN_POINT('Ctrl Pts',(-183.884539221333,-95.4948925040621,
-1.2568729675859));
#29007=CARTESIAN_POINT('Ctrl Pts',(-183.933756424313,-95.4370013790296,
-1.38512586819768));
#29008=CARTESIAN_POINT('Ctrl Pts',(-183.987818272335,-95.3732923838696,
-1.50869724720684));
#29009=CARTESIAN_POINT('Ctrl Pts',(-184.034246838454,-95.3185788029926,
-1.61482092130545));
#29010=CARTESIAN_POINT('Ctrl Pts',(-184.084247981211,-95.259574924401,-1.71749225159379));
#29011=CARTESIAN_POINT('Ctrl Pts',(-184.13715259088,-95.1970311559832,-1.81736427105629));
#29012=CARTESIAN_POINT('Ctrl Pts',(-184.139376756947,-95.1944017494282,
-1.82156299699304));
#29013=CARTESIAN_POINT('Ctrl Pts',(-184.141605799135,-95.1917663849156,
-1.82575598533418));
#29014=CARTESIAN_POINT('Ctrl Pts',(-184.143839671123,-95.1891251153873,
-1.82994324507604));
#29015=CARTESIAN_POINT('Ctrl Pts',(-184.220435087611,-95.098560776594,-1.97351678265353));
#29016=CARTESIAN_POINT('Ctrl Pts',(-184.302651756358,-95.0011215960924,
-2.11025363025844));
#29017=CARTESIAN_POINT('Ctrl Pts',(-184.388592842741,-94.898977142677,-2.24059233765731));
#29018=CARTESIAN_POINT('Ctrl Pts',(-184.433674618534,-94.8453956307228,
-2.30896359791739));
#29019=CARTESIAN_POINT('Ctrl Pts',(-184.479780684922,-94.7905200050719,
-2.37557437687181));
#29020=CARTESIAN_POINT('Ctrl Pts',(-184.526633468334,-94.73466773982,-2.4404886208611));
#29021=CARTESIAN_POINT('Ctrl Pts',(-184.527176884216,-94.7340199446255,
-2.44124152023089));
#29022=CARTESIAN_POINT('Ctrl Pts',(-184.527720426209,-94.7333719875324,
-2.44199422515958));
#29023=CARTESIAN_POINT('Ctrl Pts',(-184.528264094033,-94.7327238688657,
-2.44274673570745));
#29024=CARTESIAN_POINT('Ctrl Pts',(-184.612107889473,-94.6327717905154,
-2.55879800396048));
#29025=CARTESIAN_POINT('Ctrl Pts',(-184.69886411786,-94.5290729414887,-2.67012237576756));
#29026=CARTESIAN_POINT('Ctrl Pts',(-184.787618496314,-94.4226767227031,
-2.77711763958086));
#29027=CARTESIAN_POINT('Ctrl Pts',(-184.843651702179,-94.3555057128406,
-2.84466684389354));
#29028=CARTESIAN_POINT('Ctrl Pts',(-184.90048179645,-94.2872589546782,-2.91048943974378));
#29029=CARTESIAN_POINT('Ctrl Pts',(-184.957878667389,-94.2181996013897,
-2.9746750548167));
#29030=CARTESIAN_POINT('Ctrl Pts',(-184.958832137028,-94.2170523960528,
-2.97574129822416));
#29031=CARTESIAN_POINT('Ctrl Pts',(-184.959785764468,-94.2159049647762,
-2.9768070912445));
#29032=CARTESIAN_POINT('Ctrl Pts',(-184.960739548435,-94.2147573090282,
-2.97787243402948));
#29033=CARTESIAN_POINT('Ctrl Pts',(-185.055656879252,-94.1005465190806,
-3.08389171833809));
#29034=CARTESIAN_POINT('Ctrl Pts',(-185.152073064151,-93.9841796856407,
-3.18543351709792));
#29035=CARTESIAN_POINT('Ctrl Pts',(-185.249698961493,-93.8659730207856,
-3.28323031733737));
#29036=CARTESIAN_POINT('Ctrl Pts',(-185.303685810653,-93.8006050645476,
-3.33731167532267));
#29037=CARTESIAN_POINT('Ctrl Pts',(-185.358042346536,-93.734674788487,-3.39024870455163));
#29038=CARTESIAN_POINT('Ctrl Pts',(-185.412717994685,-93.6682377807508,
-3.44217144691258));
#29039=CARTESIAN_POINT('Ctrl Pts',(-185.414020826092,-93.6666546953517,
-3.44340868107037));
#29040=CARTESIAN_POINT('Ctrl Pts',(-185.415323838326,-93.6650713226774,
-3.44464533868886));
#29041=CARTESIAN_POINT('Ctrl Pts',(-185.41662703075,-93.6634876634248,-3.44588142160717));
#29042=CARTESIAN_POINT('Ctrl Pts',(-185.541105647225,-93.5122193555825,
-3.56394985779942));
#29043=CARTESIAN_POINT('Ctrl Pts',(-185.667207249309,-93.358359529924,-3.6768454970486));
#29044=CARTESIAN_POINT('Ctrl Pts',(-185.794631041937,-93.20222798354,-3.78530063865651));
#29045=CARTESIAN_POINT('Ctrl Pts',(-185.824114143369,-93.1661025306417,
-3.81039480572569));
#29046=CARTESIAN_POINT('Ctrl Pts',(-185.853667976554,-93.1298555283609,
-3.83525145044411));
#29047=CARTESIAN_POINT('Ctrl Pts',(-185.883288723287,-93.0934910595899,
-3.85988000049324));
#29048=CARTESIAN_POINT('Ctrl Pts',(-185.946688598849,-93.0156570057842,
-3.91259464075803));
#29049=CARTESIAN_POINT('Ctrl Pts',(-186.010647756309,-92.936973960331,-3.96446937120499));
#29050=CARTESIAN_POINT('Ctrl Pts',(-186.074793299048,-92.8578933698295,
-4.01531677064043));
#29051=CARTESIAN_POINT('Ctrl Pts',(-186.144322045734,-92.7721762005619,
-4.070431371032));
#29052=CARTESIAN_POINT('Ctrl Pts',(-186.214069607494,-92.6859919969263,
-4.12433927420305));
#29053=CARTESIAN_POINT('Ctrl Pts',(-186.283549979849,-92.5999389434393,
-4.17685870024448));
#29054=CARTESIAN_POINT('Ctrl Pts',(-186.309404272347,-92.5679178022194,
-4.19640166693666));
#29055=CARTESIAN_POINT('Ctrl Pts',(-186.335221478964,-92.5359150334324,
-4.21575288020181));
#29056=CARTESIAN_POINT('Ctrl Pts',(-186.360976297731,-92.5039621495615,
-4.23490456548554));
#29057=CARTESIAN_POINT('Ctrl Pts',(-186.362273299024,-92.5023530164482,
-4.23586903589422));
#29058=CARTESIAN_POINT('Ctrl Pts',(-186.363570144303,-92.5007440073944,
-4.23683299281394));
#29059=CARTESIAN_POINT('Ctrl Pts',(-186.364866830462,-92.4991351263001,
-4.23779643485467));
#29060=CARTESIAN_POINT('Ctrl Pts',(-186.592435857374,-92.2167757422467,
-4.40688096332591));
#29061=CARTESIAN_POINT('Ctrl Pts',(-186.821641388606,-91.9302462495062,
-4.56497378064983));
#29062=CARTESIAN_POINT('Ctrl Pts',(-187.051828931819,-91.6402373813893,
-4.71444402500823));
#29063=CARTESIAN_POINT('Ctrl Pts',(-187.144372893419,-91.5236430202006,
-4.77453662759256));
#29064=CARTESIAN_POINT('Ctrl Pts',(-187.237075726216,-91.4064860720515,
-4.83323496705587));
#29065=CARTESIAN_POINT('Ctrl Pts',(-187.3298954364,-91.2888106578876,-4.89069088055909));
#29066=CARTESIAN_POINT('Ctrl Pts',(-187.601053998392,-90.9450399649696,
-5.05853952878842));
#29067=CARTESIAN_POINT('Ctrl Pts',(-187.873240567925,-90.5968104926114,
-5.21569175079462));
#29068=CARTESIAN_POINT('Ctrl Pts',(-188.145873603651,-90.2447077922517,
-5.36433722168423));
#29069=CARTESIAN_POINT('Ctrl Pts',(-188.200938440812,-90.1735921337697,
-5.39435977059362));
#29070=CARTESIAN_POINT('Ctrl Pts',(-188.256021524338,-90.1023184107007,
-5.4240351428556));
#29071=CARTESIAN_POINT('Ctrl Pts',(-188.311118109849,-90.0308913574651,
-5.4533811546917));
#29072=CARTESIAN_POINT('Origin',(-192.01137155147,93.4192711577907,5.31766757925036));
#29073=CARTESIAN_POINT('Origin',(-192.27014422543,-93.0847597593693,-5.4533811546917));
#29074=CARTESIAN_POINT('Origin',(0.,-222.,0.));
#29075=CARTESIAN_POINT('',(199.738310248729,-222.,15.));
#29076=CARTESIAN_POINT('Origin',(199.738310248729,-222.,0.));
#29077=CARTESIAN_POINT('',(0.,-222.,15.));
#29078=CARTESIAN_POINT('Origin',(199.738310248729,222.,0.));
#29079=CARTESIAN_POINT('',(199.738310248729,222.,-15.));
#29080=CARTESIAN_POINT('',(199.738310248729,222.,-15.));
#29081=CARTESIAN_POINT('Origin',(199.738310248729,222.,0.));
#29082=CARTESIAN_POINT('Origin',(199.738310248729,-222.,0.));
#29083=CARTESIAN_POINT('Origin',(199.738310248729,222.,0.));
#29084=CARTESIAN_POINT('Origin',(-71.5953323638214,6.93889390390723E-15,
-26.5));
#29085=CARTESIAN_POINT('Ctrl Pts',(-188.311118109849,-90.0308913574651,
-5.4533811546917));
#29086=CARTESIAN_POINT('Ctrl Pts',(-188.753305639072,-89.4576407304613,
-5.68890283719888));
#29087=CARTESIAN_POINT('Ctrl Pts',(-189.193308928458,-88.8784819227758,
-5.90197859397969));
#29088=CARTESIAN_POINT('Ctrl Pts',(-189.63044941269,-88.2940948432694,-6.09829027438424));
#29089=CARTESIAN_POINT('Ctrl Pts',(-189.839578220121,-88.0145229952629,
-6.19220614145355));
#29090=CARTESIAN_POINT('Ctrl Pts',(-190.0480523925,-87.7337550679739,-6.2822852426851));
#29091=CARTESIAN_POINT('Ctrl Pts',(-190.255800837365,-87.4518682623278,
-6.36914968955112));
#29092=CARTESIAN_POINT('Ctrl Pts',(-190.782415688894,-86.7373224644024,
-6.58933958228109));
#29093=CARTESIAN_POINT('Ctrl Pts',(-191.30440717723,-86.0155284126311,-6.78845317883935));
#29094=CARTESIAN_POINT('Ctrl Pts',(-191.821164100696,-85.2870765363022,
-6.97149374860157));
#29095=CARTESIAN_POINT('Ctrl Pts',(-191.934392805452,-85.1274624920808,
-7.011600510003));
#29096=CARTESIAN_POINT('Ctrl Pts',(-192.047370341996,-84.9675289311489,
-7.05093558981425));
#29097=CARTESIAN_POINT('Ctrl Pts',(-192.16009053274,-84.8072822852053,-7.0895516218191));
#29098=CARTESIAN_POINT('Ctrl Pts',(-192.807135210935,-83.8874227749251,
-7.31121819137361));
#29099=CARTESIAN_POINT('Ctrl Pts',(-193.445667235945,-82.9572868867053,
-7.50949616528049));
#29100=CARTESIAN_POINT('Ctrl Pts',(-194.0750538067,-82.0173998381265,-7.68915683905057));
#29101=CARTESIAN_POINT('Ctrl Pts',(-194.665749224521,-81.13529176868,-7.85777298322919));
#29102=CARTESIAN_POINT('Ctrl Pts',(-195.248389252336,-80.2445949893091,
-8.00999044481605));
#29103=CARTESIAN_POINT('Ctrl Pts',(-195.822480593053,-79.3457729420087,
-8.14975356709067));
#29104=CARTESIAN_POINT('Ctrl Pts',(-196.650355260343,-78.0496168243568,
-8.35130049899169));
#29105=CARTESIAN_POINT('Ctrl Pts',(-197.460511393583,-76.7364778580625,
-8.52633259433118));
#29106=CARTESIAN_POINT('Ctrl Pts',(-198.252078897448,-75.4069267272506,
-8.68064281764092));
#29107=CARTESIAN_POINT('Ctrl Pts',(-198.594293956822,-74.8321274625641,
-8.74735510935841));
#29108=CARTESIAN_POINT('Ctrl Pts',(-198.933034987134,-74.2542612642923,
-8.81019436709263));
#29109=CARTESIAN_POINT('Ctrl Pts',(-199.268233060988,-73.6733769315866,
-8.86962868621838));
#29110=CARTESIAN_POINT('Ctrl Pts',(-199.712997529187,-72.9026185905557,
-8.94849033668896));
#29111=CARTESIAN_POINT('Ctrl Pts',(-200.151407978414,-72.1267399572591,
-9.02126337332997));
#29112=CARTESIAN_POINT('Ctrl Pts',(-200.583013021259,-71.3464384503323,
-9.08858769280887));
#29113=CARTESIAN_POINT('Ctrl Pts',(-201.014366027992,-70.5665926010997,
-9.15587269819712));
#29114=CARTESIAN_POINT('Ctrl Pts',(-201.438921493303,-69.7823291719526,
-9.21771534813081));
#29115=CARTESIAN_POINT('Ctrl Pts',(-201.85627383329,-68.9943705560089,-9.27475441892738));
#29116=CARTESIAN_POINT('Ctrl Pts',(-202.064023488162,-68.6021405028104,
-9.30314732855517));
#29117=CARTESIAN_POINT('Ctrl Pts',(-202.269989024108,-68.208995232856,-9.33034998358936));
#29118=CARTESIAN_POINT('Ctrl Pts',(-202.474124665087,-67.8150261129094,
-9.35644117223032));
#29119=CARTESIAN_POINT('Ctrl Pts',(-203.170724791756,-66.470631094265,-9.44547572408601));
#29120=CARTESIAN_POINT('Ctrl Pts',(-203.846736462659,-65.1152688211963,
-9.52164011411435));
#29121=CARTESIAN_POINT('Ctrl Pts',(-204.502059883097,-63.7490221183761,
-9.58726396269712));
#29122=CARTESIAN_POINT('Ctrl Pts',(-204.810586094828,-63.1057932845452,
-9.61815966514109));
#29123=CARTESIAN_POINT('Ctrl Pts',(-205.114526015695,-62.4601515926185,
-9.64671902957372));
#29124=CARTESIAN_POINT('Ctrl Pts',(-205.413865495665,-61.8121042464487,
-9.6731851612178));
#29125=CARTESIAN_POINT('Ctrl Pts',(-205.754227781708,-61.0752456261693,
-9.70327832858073));
#29126=CARTESIAN_POINT('Ctrl Pts',(-206.088782566592,-60.3349621177671,
-9.73065648355805));
#29127=CARTESIAN_POINT('Ctrl Pts',(-206.417157585293,-59.5920421271443,
-9.75556921716682));
#29128=CARTESIAN_POINT('Ctrl Pts',(-206.745708789431,-58.8487235322537,
-9.7804953173858));
#29129=CARTESIAN_POINT('Ctrl Pts',(-207.068073534945,-58.1027657529877,
-9.80295334994558));
#29130=CARTESIAN_POINT('Ctrl Pts',(-207.383926780309,-57.3549794466614,
-9.82319330782345));
#29131=CARTESIAN_POINT('Ctrl Pts',(-207.619735262604,-56.7967000667156,
-9.83830397652464));
#29132=CARTESIAN_POINT('Ctrl Pts',(-207.851915374644,-56.2374019541152,
-9.85217834393231));
#29133=CARTESIAN_POINT('Ctrl Pts',(-208.080349477207,-55.6774293990949,
-9.86492043799816));
#29134=CARTESIAN_POINT('Ctrl Pts',(-208.61075784454,-54.3772114135693,-9.89450670919867));
#29135=CARTESIAN_POINT('Ctrl Pts',(-209.121493376765,-53.0721049929371,
-9.91813719639479));
#29136=CARTESIAN_POINT('Ctrl Pts',(-209.61276822689,-51.7621815490425,-9.93682266532636));
#29137=CARTESIAN_POINT('Ctrl Pts',(-210.105670524664,-50.4479187178803,
-9.95557003366615));
#29138=CARTESIAN_POINT('Ctrl Pts',(-210.578983118157,-49.1288066369609,
-9.96933956672149));
#29139=CARTESIAN_POINT('Ctrl Pts',(-211.032876285271,-47.8048887258006,
-9.9791521086454));
#29140=CARTESIAN_POINT('Ctrl Pts',(-211.488405566466,-46.4761985887213,
-9.98900002109079));
#29141=CARTESIAN_POINT('Ctrl Pts',(-211.924375291595,-45.1426676490755,
-9.99486236406205));
#29142=CARTESIAN_POINT('Ctrl Pts',(-212.340911477666,-43.8043148655557,
-9.99777106082963));
#29143=CARTESIAN_POINT('Ctrl Pts',(-212.406256152434,-43.5943589714763,
-9.99822736654959));
#29144=CARTESIAN_POINT('Ctrl Pts',(-212.471122470112,-43.3842843658794,
-9.99861098248156));
#29145=CARTESIAN_POINT('Ctrl Pts',(-212.535510811764,-43.1740910731707,
-9.99892589262986));
#29146=CARTESIAN_POINT('Ctrl Pts',(-212.953022228768,-41.8111409298332,
-10.0009678551789));
#29147=CARTESIAN_POINT('Ctrl Pts',(-213.350438023984,-40.4432108877624,
-10.0000719408692));
#29148=CARTESIAN_POINT('Ctrl Pts',(-213.727826864813,-39.0703218294651,
-9.99695058699469));
#29149=CARTESIAN_POINT('Ctrl Pts',(-214.122785598877,-37.6335158993145,
-9.99368391389394));
#29150=CARTESIAN_POINT('Ctrl Pts',(-214.495809725065,-36.1912782559092,
-9.98797976034421));
#29151=CARTESIAN_POINT('Ctrl Pts',(-214.84691994715,-34.7436137410651,-9.98065477386882));
#29152=CARTESIAN_POINT('Ctrl Pts',(-215.198030169234,-33.295949226221,-9.97332978739343));
#29153=CARTESIAN_POINT('Ctrl Pts',(-215.527226576327,-31.8428574725277,
-9.96438396799237));
#29154=CARTESIAN_POINT('Ctrl Pts',(-215.834469144665,-30.3843292117711,
-9.95463396318898));
#29155=CARTESIAN_POINT('Ctrl Pts',(-216.12479711533,-29.006097177089,-9.94542072452923));
#29156=CARTESIAN_POINT('Ctrl Pts',(-216.395519847526,-27.6230191217557,
-9.93547880367801));
#29157=CARTESIAN_POINT('Ctrl Pts',(-216.646556008205,-26.235063563848,-9.9252656029735));
#29158=CARTESIAN_POINT('Ctrl Pts',(-216.897054662457,-24.8500798289305,
-9.91507427027801));
#29159=CARTESIAN_POINT('Ctrl Pts',(-217.127950993222,-23.4602391649776,
-9.904612818188));
#29160=CARTESIAN_POINT('Ctrl Pts',(-217.339112418497,-22.0655073883797,
-9.89433571722511));
#29161=CARTESIAN_POINT('Ctrl Pts',(-217.549435266681,-20.6763144554178,
-9.88409942931046));
#29162=CARTESIAN_POINT('Ctrl Pts',(-217.740179653031,-19.2822688917432,
-9.8740460312175));
#29163=CARTESIAN_POINT('Ctrl Pts',(-217.911162846412,-17.8833383662589,
-9.86462460047875));
#29164=CARTESIAN_POINT('Ctrl Pts',(-217.93455057477,-17.6919873540601,-9.86333590152238));
#29165=CARTESIAN_POINT('Ctrl Pts',(-217.957568495531,-17.500544951324,-9.86205902655124));
#29166=CARTESIAN_POINT('Ctrl Pts',(-217.980216065289,-17.3090110820993,
-9.86079512484355));
#29167=CARTESIAN_POINT('Ctrl Pts',(-218.144483248337,-15.9197790588204,
-9.85162780245975));
#29168=CARTESIAN_POINT('Ctrl Pts',(-218.289319103681,-14.5252556083932,
-9.84310086102437));
#29169=CARTESIAN_POINT('Ctrl Pts',(-218.414393171551,-13.1262875356464,
-9.83550018779937));
#29170=CARTESIAN_POINT('Ctrl Pts',(-218.487680928573,-12.3065554045771,
-9.831046536439));
#29171=CARTESIAN_POINT('Ctrl Pts',(-218.55418451901,-11.4852976098094,-9.82691091286767));
#29172=CARTESIAN_POINT('Ctrl Pts',(-218.613845276764,-10.6626873629055,
-9.82315083289945));
#29173=CARTESIAN_POINT('Ctrl Pts',(-218.714243156394,-9.2783884089601,-9.81682332265223));
#29174=CARTESIAN_POINT('Ctrl Pts',(-218.794867940585,-7.89578614496809,
-9.8115860039582));
#29175=CARTESIAN_POINT('Ctrl Pts',(-218.855960361108,-6.51486629004492,
-9.80756307330259));
#29176=CARTESIAN_POINT('Ctrl Pts',(-218.893128271323,-5.67473088955579,
-9.8051155696003));
#29177=CARTESIAN_POINT('Ctrl Pts',(-218.923065578444,-4.83521786741106,
-9.80311755493369));
#29178=CARTESIAN_POINT('Ctrl Pts',(-218.945817455584,-3.99632132774656,
-9.80159699667983));
#29179=CARTESIAN_POINT('Ctrl Pts',(-218.984176164557,-2.58197700676585,
-9.79903339934764));
#29180=CARTESIAN_POINT('Ctrl Pts',(-219.002113407906,-1.16938036292585,
-9.79787591200204));
#29181=CARTESIAN_POINT('Ctrl Pts',(-218.999802216758,0.241471131014165,
-9.79806426229321));
#29182=CARTESIAN_POINT('Ctrl Pts',(-218.997485328933,1.65580012391016,-9.79825307683448));
#29183=CARTESIAN_POINT('Ctrl Pts',(-218.974820086377,3.06837564753467,-9.7997943716916));
#29184=CARTESIAN_POINT('Ctrl Pts',(-218.931929074689,4.47920870148126,-9.80262742773335));
#29185=CARTESIAN_POINT('Ctrl Pts',(-218.888937672361,5.89334394924374,-9.80546711482199));
#29186=CARTESIAN_POINT('Ctrl Pts',(-218.825625720191,7.30572885744436,-9.80960461716078));
#29187=CARTESIAN_POINT('Ctrl Pts',(-218.742064526062,8.71637854307249,-9.81497878826245));
#29188=CARTESIAN_POINT('Ctrl Pts',(-218.731349327016,8.89726863592627,-9.81566792768488));
#29189=CARTESIAN_POINT('Ctrl Pts',(-218.720301091681,9.07813019772746,-9.81637740212719));
#29190=CARTESIAN_POINT('Ctrl Pts',(-218.708919908478,9.25896326123478,-9.81710708265811));
#29191=CARTESIAN_POINT('Ctrl Pts',(-218.619563682027,10.6787242724598,-9.8228359684512));
#29192=CARTESIAN_POINT('Ctrl Pts',(-218.509688811122,12.0967197729986,-9.8298080272327));
#29193=CARTESIAN_POINT('Ctrl Pts',(-218.379310061933,13.5129542311266,-9.83770685533299));
#29194=CARTESIAN_POINT('Ctrl Pts',(-218.242405787213,15.0000719748565,-9.84600102396813));
#29195=CARTESIAN_POINT('Ctrl Pts',(-218.0828942667,16.4852483906094,-9.8553170541224));
#29196=CARTESIAN_POINT('Ctrl Pts',(-217.900731068501,17.9684821506137,-9.86528861611505));
#29197=CARTESIAN_POINT('Ctrl Pts',(-217.718567870302,19.451715910618,-9.8752601781077));
#29198=CARTESIAN_POINT('Ctrl Pts',(-217.513752947392,20.9330073981508,-9.88588727193872));
#29199=CARTESIAN_POINT('Ctrl Pts',(-217.286179447546,22.4123429600545,-9.89680356792739));
#29200=CARTESIAN_POINT('Ctrl Pts',(-217.074537568303,23.7881154404372,-9.90695565241428));
#29201=CARTESIAN_POINT('Ctrl Pts',(-216.843213111179,25.1621874059895,-9.91736416322261));
#29202=CARTESIAN_POINT('Ctrl Pts',(-216.592066415917,26.5345652905463,-9.92749162982048));
#29203=CARTESIAN_POINT('Ctrl Pts',(-216.341668290249,27.9028526559885,-9.93758891042062));
#29204=CARTESIAN_POINT('Ctrl Pts',(-216.071565840309,29.2694562987497,-9.94740681967818));
#29205=CARTESIAN_POINT('Ctrl Pts',(-215.781572186617,30.6343644735032,-9.95641267871605));
#29206=CARTESIAN_POINT('Ctrl Pts',(-215.493060155512,31.9922991205487,-9.96537252542233));
#29207=CARTESIAN_POINT('Ctrl Pts',(-215.184859557881,33.3485558414738,-9.97352859849281));
#29208=CARTESIAN_POINT('Ctrl Pts',(-214.856739636078,34.703101119423,-9.98035634202435));
#29209=CARTESIAN_POINT('Ctrl Pts',(-214.795334533757,34.9565937782491,-9.9816341013505));
#29210=CARTESIAN_POINT('Ctrl Pts',(-214.733231682609,35.2100264299969,-9.98286533962214));
#29211=CARTESIAN_POINT('Ctrl Pts',(-214.670429391573,35.4633987574771,-9.98404661882751));
#29212=CARTESIAN_POINT('Ctrl Pts',(-214.359497476236,36.7178361637757,-9.98989509027358));
#29213=CARTESIAN_POINT('Ctrl Pts',(-214.032421066029,37.9667411686325,-9.99445006270918));
#29214=CARTESIAN_POINT('Ctrl Pts',(-213.689538210722,39.2093446217989,-9.99716936427343));
#29215=CARTESIAN_POINT('Ctrl Pts',(-213.440231444473,40.1128294238039,-9.99914654181073));
#29216=CARTESIAN_POINT('Ctrl Pts',(-213.182569462386,41.0129832213348,-10.0001532732747));
#29217=CARTESIAN_POINT('Ctrl Pts',(-212.916698050239,41.9095173135889,-9.99998115667634));
#29218=CARTESIAN_POINT('Ctrl Pts',(-212.509602595805,43.2822672108238,-9.99971761617662));
#29219=CARTESIAN_POINT('Ctrl Pts',(-212.083102729471,44.647086672049,-9.99669713415972));
#29220=CARTESIAN_POINT('Ctrl Pts',(-211.63735202868,46.004008185371,-9.99003728668321));
#29221=CARTESIAN_POINT('Ctrl Pts',(-211.391599599651,46.752109662965,-9.98636556235074));
#29222=CARTESIAN_POINT('Ctrl Pts',(-211.139994833097,47.4978104022167,-9.98158762888982));
#29223=CARTESIAN_POINT('Ctrl Pts',(-210.882556783091,48.2411147726525,-9.9755556113417));
#29224=CARTESIAN_POINT('Ctrl Pts',(-210.407166434106,49.6137157694966,-9.96441676482224));
#29225=CARTESIAN_POINT('Ctrl Pts',(-209.911886250968,50.9781493632379,-9.9491269391516));
#29226=CARTESIAN_POINT('Ctrl Pts',(-209.396804182012,52.3344093849598,-9.92839606297258));
#29227=CARTESIAN_POINT('Ctrl Pts',(-208.869479898179,53.7229043214992,-9.90717246562135));
#29228=CARTESIAN_POINT('Ctrl Pts',(-208.321401349102,55.1028329191272,-9.88024610376969));
#29229=CARTESIAN_POINT('Ctrl Pts',(-207.752608950314,56.4741717378989,-9.84623271715167));
#29230=CARTESIAN_POINT('Ctrl Pts',(-207.183816551525,57.8455105566706,-9.81221933053365));
#29231=CARTESIAN_POINT('Ctrl Pts',(-206.594310169254,59.2082599190967,-9.77111891914926));
#29232=CARTESIAN_POINT('Ctrl Pts',(-205.984077548804,60.5623745285646,-9.72154722273255));
#29233=CARTESIAN_POINT('Ctrl Pts',(-205.383262636071,61.8955911145903,-9.6727405653063));
#29234=CARTESIAN_POINT('Ctrl Pts',(-204.76235657447,63.2204360342108,-9.61598017611668));
#29235=CARTESIAN_POINT('Ctrl Pts',(-204.121307325464,64.536826706914,-9.54877517923461));
#29236=CARTESIAN_POINT('Ctrl Pts',(-203.472743362976,65.8686487973313,-9.48078237034439));
#29237=CARTESIAN_POINT('Ctrl Pts',(-202.803561129253,67.1918176216725,-9.40209864421725));
#29238=CARTESIAN_POINT('Ctrl Pts',(-202.11366114301,68.5062179193968,-9.31014449600325));
#29239=CARTESIAN_POINT('Ctrl Pts',(-201.423761156767,69.8206182171212,-9.21819034778924));
#29240=CARTESIAN_POINT('Ctrl Pts',(-200.713143257863,71.1262502867284,-9.11296577748836));
#29241=CARTESIAN_POINT('Ctrl Pts',(-199.981664414448,72.4229644761836,-8.99189128025066));
#29242=CARTESIAN_POINT('Ctrl Pts',(-199.6776144015,72.961962930674,-8.94156487261202));
#29243=CARTESIAN_POINT('Ctrl Pts',(-199.369834898682,73.4996320589593,-8.88837986748052));
#29244=CARTESIAN_POINT('Ctrl Pts',(-199.058853023589,74.0350386097636,-8.83213170660312));
#29245=CARTESIAN_POINT('Ctrl Pts',(-198.810885502973,74.4619555639597,-8.78728112813178));
#29246=CARTESIAN_POINT('Ctrl Pts',(-198.560882815212,74.8874344426336,-8.74048300008057));
#29247=CARTESIAN_POINT('Ctrl Pts',(-198.30913267803,75.3110141404511,-8.69163361829107));
#29248=CARTESIAN_POINT('Ctrl Pts',(-197.74165679773,76.2658150576885,-8.58152108272949));
#29249=CARTESIAN_POINT('Ctrl Pts',(-197.164705398621,77.2119850731197,-8.46091798763827));
#29250=CARTESIAN_POINT('Ctrl Pts',(-196.578625312678,78.1492963793824,-8.32767843937961));
#29251=CARTESIAN_POINT('Ctrl Pts',(-195.949038803721,79.1561870198767,-8.18454813337673));
#29252=CARTESIAN_POINT('Ctrl Pts',(-195.308874570202,80.1529188927709,-8.02725639835802));
#29253=CARTESIAN_POINT('Ctrl Pts',(-194.658762385835,81.1389439920761,-7.85130852010962));
#29254=CARTESIAN_POINT('Ctrl Pts',(-194.098499825935,81.9886941729618,-7.69967775384069));
#29255=CARTESIAN_POINT('Ctrl Pts',(-193.530849705582,82.8304930966393,-7.53419128798475));
#29256=CARTESIAN_POINT('Ctrl Pts',(-192.956236453638,83.6640125707261,-7.35197230730516));
#29257=CARTESIAN_POINT('Ctrl Pts',(-192.419403832868,84.442728415206,-7.18173416430839));
#29258=CARTESIAN_POINT('Ctrl Pts',(-191.876510663817,85.2141889951778,-6.99671260528906));
#29259=CARTESIAN_POINT('Ctrl Pts',(-191.328162094401,85.977819963292,-6.79234392467887));
#29260=CARTESIAN_POINT('Ctrl Pts',(-191.242507083244,86.0971032490376,-6.76042043186023));
#29261=CARTESIAN_POINT('Ctrl Pts',(-191.156719036077,86.2161955608546,-6.72802486677896));
#29262=CARTESIAN_POINT('Ctrl Pts',(-191.070800343556,86.3350947874365,-6.69513983518131));
#29263=CARTESIAN_POINT('Ctrl Pts',(-190.608513931787,86.9748333030743,-6.51820158330396));
#29264=CARTESIAN_POINT('Ctrl Pts',(-190.142422121888,87.609006867386,-6.32728225133389));
#29265=CARTESIAN_POINT('Ctrl Pts',(-189.673163685796,88.2369638600037,-6.11735698536059));
#29266=CARTESIAN_POINT('Ctrl Pts',(-189.496875586272,88.4728708491959,-6.03849356313051));
#29267=CARTESIAN_POINT('Ctrl Pts',(-189.320140977775,88.707900834228,-5.95694781816414));
#29268=CARTESIAN_POINT('Ctrl Pts',(-189.142995147248,88.9420205250928,-5.87245333700276));
#29269=CARTESIAN_POINT('Ctrl Pts',(-188.818651423809,89.3706800766031,-5.717748851165));
#29270=CARTESIAN_POINT('Ctrl Pts',(-188.49293989293,89.7962712759086,-5.55305032555424));
#29271=CARTESIAN_POINT('Ctrl Pts',(-188.166231145434,90.2184105278924,-5.37541261640281));
#29272=CARTESIAN_POINT('Ctrl Pts',(-187.941553999842,90.5087150970382,-5.25325141396333));
#29273=CARTESIAN_POINT('Ctrl Pts',(-187.716679186465,90.7970273844016,-5.12511114867476));
#29274=CARTESIAN_POINT('Ctrl Pts',(-187.492754926394,91.0819602571486,-4.99016685446453));
#29275=CARTESIAN_POINT('Ctrl Pts',(-187.391065228939,91.2113555161321,-4.92888522090169));
#29276=CARTESIAN_POINT('Ctrl Pts',(-187.289572125172,91.3400542891487,-4.86620039318761));
#29277=CARTESIAN_POINT('Ctrl Pts',(-187.188385892342,91.467928897974,-4.80203510975558));
#29278=CARTESIAN_POINT('Ctrl Pts',(-186.926482284857,91.798910894441,-4.63595402603387));
#29279=CARTESIAN_POINT('Ctrl Pts',(-186.666166588022,92.1249576589846,-4.45982540733765));
#29280=CARTESIAN_POINT('Ctrl Pts',(-186.408598112086,92.4448486891005,-4.27016769975641));
#29281=CARTESIAN_POINT('Ctrl Pts',(-186.347527747809,92.520695943571,-4.22519921031799));
#29282=CARTESIAN_POINT('Ctrl Pts',(-186.286612000581,92.5961972877401,-4.17947014218683));
#29283=CARTESIAN_POINT('Ctrl Pts',(-186.225866640945,92.6713367351173,-4.13293408803839));
#29284=CARTESIAN_POINT('Ctrl Pts',(-186.010419293658,92.9378360152417,-3.96788330095816));
#29285=CARTESIAN_POINT('Ctrl Pts',(-185.797040930281,93.1998680077896,-3.79291563167685));
#29286=CARTESIAN_POINT('Ctrl Pts',(-185.587151181677,93.4558788066831,-3.60367209755208));
#29287=CARTESIAN_POINT('Ctrl Pts',(-185.488273569283,93.576483727648,-3.5145207743467));
#29288=CARTESIAN_POINT('Ctrl Pts',(-185.390170766711,93.6957528796746,-3.4222012268844));
#29289=CARTESIAN_POINT('Ctrl Pts',(-185.292994175947,93.8135264201691,-3.32625772752428));
#29290=CARTESIAN_POINT('Ctrl Pts',(-185.162032493132,93.9722459320697,-3.19695784128052));
#29291=CARTESIAN_POINT('Ctrl Pts',(-185.032274848444,94.1288222169724,-3.0606810953648));
#29292=CARTESIAN_POINT('Ctrl Pts',(-184.905880009225,94.2807288539447,-2.91629164267507));
#29293=CARTESIAN_POINT('Ctrl Pts',(-184.773357322611,94.4400001957996,-2.7649019316134));
#29294=CARTESIAN_POINT('Ctrl Pts',(-184.644531572858,94.5941382067379,-2.60459380798681));
#29295=CARTESIAN_POINT('Ctrl Pts',(-184.52193501311,94.7402683921781,-2.43405808220338));
#29296=CARTESIAN_POINT('Ctrl Pts',(-184.490522330022,94.777711051371,-2.39036203787495));
#29297=CARTESIAN_POINT('Ctrl Pts',(-184.459518816605,94.8146281515711,-2.34599452244704));
#29298=CARTESIAN_POINT('Ctrl Pts',(-184.42896747061,94.8509716846399,-2.30093351259949));
#29299=CARTESIAN_POINT('Ctrl Pts',(-184.312740025998,94.9892345283602,-2.12950649831777));
#29300=CARTESIAN_POINT('Ctrl Pts',(-184.202585838296,95.1197493985745,-1.94735170602647));
#29301=CARTESIAN_POINT('Ctrl Pts',(-184.102034801778,95.2385318422614,-1.74979548300606));
#29302=CARTESIAN_POINT('Ctrl Pts',(-184.088602492028,95.2543996307167,-1.72340454291751));
#29303=CARTESIAN_POINT('Ctrl Pts',(-184.075341611869,95.2700580979542,-1.6967387568678));
#29304=CARTESIAN_POINT('Ctrl Pts',(-184.062260624235,95.2854977874351,-1.66978698322322));
#29305=CARTESIAN_POINT('Ctrl Pts',(-183.951258512844,95.4165152747594,-1.44108072159684));
#29306=CARTESIAN_POINT('Ctrl Pts',(-183.856402416991,95.5280069404102,-1.19842060958046));
#29307=CARTESIAN_POINT('Ctrl Pts',(-183.78559008165,95.6110982791194,-0.935265073867139));
#29308=CARTESIAN_POINT('Ctrl Pts',(-183.75018391398,95.6526439484739,-0.803687306010473));
#29309=CARTESIAN_POINT('Ctrl Pts',(-183.720972654883,95.6868740766621,-0.666464316175631));
#29310=CARTESIAN_POINT('Ctrl Pts',(-183.700029885832,95.711403889144,-0.528231852282087));
#29311=CARTESIAN_POINT('Ctrl Pts',(-183.67908711678,95.7359337016259,-0.389999388388542));
#29312=CARTESIAN_POINT('Ctrl Pts',(-183.666054681306,95.7511842509038,-0.249647095948257));
#29313=CARTESIAN_POINT('Ctrl Pts',(-183.66168335083,95.7563001446319,-0.106977127421175));
#29314=CARTESIAN_POINT('Ctrl Pts',(-183.657312020355,95.7614160383599,0.0356928411059037));
#29315=CARTESIAN_POINT('Ctrl Pts',(-183.661865337804,95.7560891876555,0.179679148990217));
#29316=CARTESIAN_POINT('Ctrl Pts',(-183.674665679525,95.7411044663663,0.319496061024171));
#29317=CARTESIAN_POINT('Ctrl Pts',(-183.687466021247,95.7261197450771,0.459312973058134));
#29318=CARTESIAN_POINT('Ctrl Pts',(-183.708428755956,95.7015755681125,0.596571383448631));
#29319=CARTESIAN_POINT('Ctrl Pts',(-183.73677770673,95.6683452210586,0.731509051287532));
#29320=CARTESIAN_POINT('Ctrl Pts',(-183.765126657504,95.6351148740048,0.866446719126424));
#29321=CARTESIAN_POINT('Ctrl Pts',(-183.801164672152,95.5928412644945,0.999673886209484));
#29322=CARTESIAN_POINT('Ctrl Pts',(-183.842486096339,95.544296113797,1.12685895415084));
#29323=CARTESIAN_POINT('Ctrl Pts',(-183.883807520525,95.4957509630995,1.25404402209221));
#29324=CARTESIAN_POINT('Ctrl Pts',(-183.930563125213,95.4407576673987,1.37625930381363));
#29325=CARTESIAN_POINT('Ctrl Pts',(-183.981732092056,95.3804654898362,1.49441051952705));
#29326=CARTESIAN_POINT('Ctrl Pts',(-184.05777694133,95.2908621650469,1.67000115472771));
#29327=CARTESIAN_POINT('Ctrl Pts',(-184.143477886773,95.189658168371,1.83625903517367));
#29328=CARTESIAN_POINT('Ctrl Pts',(-184.234795490352,95.0814776257665,1.99288757663377));
#29329=CARTESIAN_POINT('Ctrl Pts',(-184.266369245604,95.044073381225,2.04704308487863));
#29330=CARTESIAN_POINT('Ctrl Pts',(-184.298614785763,95.0058353815126,2.10004742185922));
#29331=CARTESIAN_POINT('Ctrl Pts',(-184.331366318257,94.9669557749258,2.15188832834384));
#29332=CARTESIAN_POINT('Ctrl Pts',(-184.458841821245,94.8156285841579,2.35366348591041));
#29333=CARTESIAN_POINT('Ctrl Pts',(-184.595169875239,94.653167207116,2.54014556267795));
#29334=CARTESIAN_POINT('Ctrl Pts',(-184.737488050318,94.4827425911459,2.71592585637909));
#29335=CARTESIAN_POINT('Ctrl Pts',(-184.85791892067,94.3385278074816,2.86467266084904));
#29336=CARTESIAN_POINT('Ctrl Pts',(-184.982907743565,94.1882878961831,3.00586283997828));
#29337=CARTESIAN_POINT('Ctrl Pts',(-185.110153711901,94.0346817681954,3.13988186032778));
#29338=CARTESIAN_POINT('Ctrl Pts',(-185.133279603762,94.0067651375047,3.16423869781617));
#29339=CARTESIAN_POINT('Ctrl Pts',(-185.156480155079,93.9787374103966,3.18835867174178));
#29340=CARTESIAN_POINT('Ctrl Pts',(-185.179741698894,93.9506146703416,3.21224409603392));
#29341=CARTESIAN_POINT('Ctrl Pts',(-185.375067641756,93.714469521897,3.4128087299952));
#29342=CARTESIAN_POINT('Ctrl Pts',(-185.57531853868,93.470864259905,3.59807650580166));
#29343=CARTESIAN_POINT('Ctrl Pts',(-185.778946495124,93.2214476654712,3.7719301043373));
#29344=CARTESIAN_POINT('Ctrl Pts',(-185.890683969115,93.0845844335245,3.86732939176304));
#29345=CARTESIAN_POINT('Ctrl Pts',(-186.003438949569,92.9459719373273,3.95929177436257));
#29346=CARTESIAN_POINT('Ctrl Pts',(-186.116960759486,92.8058870467681,4.04845878075692));
#29347=CARTESIAN_POINT('Ctrl Pts',(-186.336052281991,92.5355300821047,4.2205467275774));
#29348=CARTESIAN_POINT('Ctrl Pts',(-186.556974212558,92.2609504033717,4.38110940427998));
#29349=CARTESIAN_POINT('Ctrl Pts',(-186.778501492463,91.9835506512719,4.53240916560392));
#29350=CARTESIAN_POINT('Ctrl Pts',(-186.880937788642,91.8552783988506,4.60237159718119));
#29351=CARTESIAN_POINT('Ctrl Pts',(-186.983504074352,91.7264036161273,4.67035340948399));
#29352=CARTESIAN_POINT('Ctrl Pts',(-187.086082139975,91.5970674043341,4.73657828946882));
#29353=CARTESIAN_POINT('Ctrl Pts',(-187.410494074091,91.1880305370078,4.94602015476302));
#29354=CARTESIAN_POINT('Ctrl Pts',(-187.735717460477,90.7735000599875,5.13817049334406));
#29355=CARTESIAN_POINT('Ctrl Pts',(-188.06083509298,90.3544283086145,5.31766757924143));
#29356=CARTESIAN_POINT('Ctrl Pts',(-188.145233520197,90.2455348162912,5.3635191399407));
#29357=CARTESIAN_POINT('Ctrl Pts',(-187.854664851553,90.6205738707536,6.83263373170868));
#29358=CARTESIAN_POINT('Ctrl Pts',(-188.302848962895,91.4632161367811,8.04608569871648));
#29359=CARTESIAN_POINT('Ctrl Pts',(-187.791407151483,90.7024945656512,5.17051448656997));
#29360=CARTESIAN_POINT('Ctrl Pts',(-187.496540276221,91.0800720173262,6.57808105135662));
#29361=CARTESIAN_POINT('Ctrl Pts',(-187.88687547988,91.8985142221956,7.75653201531377));
#29362=CARTESIAN_POINT('Ctrl Pts',(-187.437220699584,91.1543549984681,4.9629292066438));
#29363=CARTESIAN_POINT('Ctrl Pts',(-187.136870690502,91.5359208617972,6.30546516147755));
#29364=CARTESIAN_POINT('Ctrl Pts',(-187.47070368759,92.3280722645737,7.44513708416162));
#29365=CARTESIAN_POINT('Ctrl Pts',(-186.758422149138,92.0101784299077,4.52454213939994));
#29366=CARTESIAN_POINT('Ctrl Pts',(-186.447354126494,92.3993958986497,5.73365867686477));
#29367=CARTESIAN_POINT('Ctrl Pts',(-186.673417663121,93.1401290348249,6.78749067092915));
#29368=CARTESIAN_POINT('Ctrl Pts',(-186.432985631702,92.4159647578489,4.29662116512001));
#29369=CARTESIAN_POINT('Ctrl Pts',(-186.116813727194,92.8087490972247,5.43831752668723));
#29370=CARTESIAN_POINT('Ctrl Pts',(-186.291328581577,93.5244589650537,6.44557505453847));
#29371=CARTESIAN_POINT('Ctrl Pts',(-185.789504878419,93.2099142476764,3.79054251520617));
#29372=CARTESIAN_POINT('Ctrl Pts',(-185.463263222825,93.6095176182921,4.78647394195717));
#29373=CARTESIAN_POINT('Ctrl Pts',(-185.53612909977,94.2750879221146,5.68638123862275));
#29374=CARTESIAN_POINT('Ctrl Pts',(-185.473492555278,93.5955608302612,3.5147156518481));
#29375=CARTESIAN_POINT('Ctrl Pts',(-185.142185731736,93.9986018940583,4.43322287886808));
#29376=CARTESIAN_POINT('Ctrl Pts',(-185.165403861164,94.6390060126994,5.27259965429573));
#29377=CARTESIAN_POINT('Ctrl Pts',(-185.016589769184,94.1478172607574,3.04374369325038));
#29378=CARTESIAN_POINT('Ctrl Pts',(-184.677473990833,94.5562789886833,3.83252013850768));
#29379=CARTESIAN_POINT('Ctrl Pts',(-184.629593327285,95.1592700205275,4.56607106412171));
#29380=CARTESIAN_POINT('Ctrl Pts',(-184.866799006187,94.3279436322682,2.87648998617678));
#29381=CARTESIAN_POINT('Ctrl Pts',(-184.52529718626,94.7379585618407,3.6200170612726));
#29382=CARTESIAN_POINT('Ctrl Pts',(-184.453967955319,95.3288078676141,4.31516546799618));
#29383=CARTESIAN_POINT('Ctrl Pts',(-184.579916698489,94.6713779749968,2.5196724298392));
#29384=CARTESIAN_POINT('Ctrl Pts',(-184.233884394348,95.0842876797572,3.16778187881883));
#29385=CARTESIAN_POINT('Ctrl Pts',(-184.117665437549,95.6517941247141,3.77988572544218));
#29386=CARTESIAN_POINT('Ctrl Pts',(-184.44239986753,94.8352001907092,2.32993307581778));
#29387=CARTESIAN_POINT('Ctrl Pts',(-184.094156916584,95.2495304257977,2.9278452901178));
#29388=CARTESIAN_POINT('Ctrl Pts',(-183.956489556471,95.8057270256804,3.49524829819147));
#29389=CARTESIAN_POINT('Ctrl Pts',(-184.185294918109,95.1402973045157,1.91734932039146));
#29390=CARTESIAN_POINT('Ctrl Pts',(-183.832981297565,95.5571842813552,2.40725694755477));
#29391=CARTESIAN_POINT('Ctrl Pts',(-183.655197053014,96.0922042485234,2.87631092236716));
#29392=CARTESIAN_POINT('Ctrl Pts',(-184.064453461112,95.2830402548575,1.69197261173593));
#29393=CARTESIAN_POINT('Ctrl Pts',(-183.710171068013,95.7011829603298,2.12341452229605));
#29394=CARTESIAN_POINT('Ctrl Pts',(-183.513612438245,96.2261237477396,2.53821212995774));
#29395=CARTESIAN_POINT('Ctrl Pts',(-183.911202264701,95.4635408941671,1.32666688325273));
#29396=CARTESIAN_POINT('Ctrl Pts',(-183.554420819748,95.8832673602713,1.66399482314503));
#29397=CARTESIAN_POINT('Ctrl Pts',(-183.334075436563,96.3953763623405,1.99019884061584));
#29398=CARTESIAN_POINT('Ctrl Pts',(-183.864744551489,95.5181608807362,1.20034832248043));
#29399=CARTESIAN_POINT('Ctrl Pts',(-183.507217373514,95.9383518302635,1.50531552343668));
#29400=CARTESIAN_POINT('Ctrl Pts',(-183.279653114889,96.4465756811072,1.80070209637048));
#29401=CARTESIAN_POINT('Ctrl Pts',(-183.783468331685,95.6136084402799,0.936341958789021));
#29402=CARTESIAN_POINT('Ctrl Pts',(-183.424650598207,96.0345934282162,1.17391428722675));
#29403=CARTESIAN_POINT('Ctrl Pts',(-183.184447352807,96.5360269050087,1.40465304838242));
#29404=CARTESIAN_POINT('Ctrl Pts',(-183.748737326012,95.654333157593,0.798204067099665));
#29405=CARTESIAN_POINT('Ctrl Pts',(-183.389359661152,96.075666167106,1.0006029019253));
#29406=CARTESIAN_POINT('Ctrl Pts',(-183.143766417956,96.5741824061768,1.1974255383652));
#29407=CARTESIAN_POINT('Ctrl Pts',(-183.695928409161,95.7162162993234,0.518880068927119));
#29408=CARTESIAN_POINT('Ctrl Pts',(-183.335711711721,96.1380633310152,0.650342007065702));
#29409=CARTESIAN_POINT('Ctrl Pts',(-183.081912119256,96.6321546625029,0.778397747287054));
#29410=CARTESIAN_POINT('Ctrl Pts',(-183.677440490251,95.7378571902513,0.376560792571389));
#29411=CARTESIAN_POINT('Ctrl Pts',(-183.316924770873,96.1598898803611,0.471927258717125));
#29412=CARTESIAN_POINT('Ctrl Pts',(-183.060258441793,96.6524237482766,0.564897533939989));
#29413=CARTESIAN_POINT('Ctrl Pts',(-183.658185995667,95.760394199856,0.0859862681696598));
#29414=CARTESIAN_POINT('Ctrl Pts',(-183.297364262565,96.1826139348272,0.107762579034491));
#29415=CARTESIAN_POINT('Ctrl Pts',(-183.037706970332,96.6735319375049,0.128992270488467));
#29416=CARTESIAN_POINT('Ctrl Pts',(-183.657681880049,95.7609839412904,-0.063896210583788));
#29417=CARTESIAN_POINT('Ctrl Pts',(-183.296852000031,96.1832087243297,-0.0800795353757084));
#29418=CARTESIAN_POINT('Ctrl Pts',(-183.037116546925,96.6740842350221,-0.0958538786891257));
#29419=CARTESIAN_POINT('Ctrl Pts',(-183.675244045363,95.7404283569817,-0.355921350698398));
#29420=CARTESIAN_POINT('Ctrl Pts',(-183.31469328487,96.162482543441,-0.44605714576703));
#29421=CARTESIAN_POINT('Ctrl Pts',(-183.057685885535,96.6548319532991,-0.533935282757487));
#29422=CARTESIAN_POINT('Ctrl Pts',(-183.693020864062,95.7196211416447,-0.499360341536995));
#29423=CARTESIAN_POINT('Ctrl Pts',(-183.33275775371,96.141496684891,-0.625871301849139));
#29424=CARTESIAN_POINT('Ctrl Pts',(-183.0785066467,96.6353439239973,-0.749115235509941));
#29425=CARTESIAN_POINT('Ctrl Pts',(-183.744901665609,95.6588299326157,-0.78155798871691));
#29426=CARTESIAN_POINT('Ctrl Pts',(-183.385462858047,96.0802005494342,-0.979723363419466));
#29427=CARTESIAN_POINT('Ctrl Pts',(-183.139273685515,96.5783953473938,-1.17245393006151));
#29428=CARTESIAN_POINT('Ctrl Pts',(-183.779175195977,95.618644870505,-0.920237396574461));
#29429=CARTESIAN_POINT('Ctrl Pts',(-183.420288799078,96.0396722809014,-1.15370660831193));
#29430=CARTESIAN_POINT('Ctrl Pts',(-183.179418644892,96.5407460179378,-1.38049379518866));
#29431=CARTESIAN_POINT('Ctrl Pts',(-183.85908515349,95.524811693759,-1.18387312000799));
#29432=CARTESIAN_POINT('Ctrl Pts',(-183.501467654743,95.9450585544367,-1.48462552841789));
#29433=CARTESIAN_POINT('Ctrl Pts',(-183.273023596524,96.4528094730268,-1.77598682731276));
#29434=CARTESIAN_POINT('Ctrl Pts',(-183.9049533987,95.4708918026245,-1.3102946528729));
#29435=CARTESIAN_POINT('Ctrl Pts',(-183.548072370971,95.8906799738278,-1.64342456925302));
#29436=CARTESIAN_POINT('Ctrl Pts',(-183.326755114843,96.4022676282472,-1.9656380451627));
#29437=CARTESIAN_POINT('Ctrl Pts',(-184.006197987058,95.3516620124118,-1.55440286313822));
#29438=CARTESIAN_POINT('Ctrl Pts',(-183.650923334156,95.7704563495827,-1.95026772005439));
#29439=CARTESIAN_POINT('Ctrl Pts',(-183.445364605803,96.2904706695442,-2.33183688685736));
#29440=CARTESIAN_POINT('Ctrl Pts',(-184.061902804819,95.2859635471583,-1.67265649549514));
#29441=CARTESIAN_POINT('Ctrl Pts',(-183.707519331346,95.7042005353516,-2.09904096749872));
#29442=CARTESIAN_POINT('Ctrl Pts',(-183.510627455621,96.2288509060907,-2.50923503171724));
#29443=CARTESIAN_POINT('Ctrl Pts',(-184.238169879718,95.07765401711,-2.01149467785066));
#29444=CARTESIAN_POINT('Ctrl Pts',(-183.886670042307,95.4940451899596,-2.52591331873638));
#29445=CARTESIAN_POINT('Ctrl Pts',(-183.717155446954,96.0334014306346,-3.017543046058));
#29446=CARTESIAN_POINT('Ctrl Pts',(-184.367342568346,94.9244689409693,-2.21657754164571));
#29447=CARTESIAN_POINT('Ctrl Pts',(-184.017930454936,95.3395258984641,-2.78467603615262));
#29448=CARTESIAN_POINT('Ctrl Pts',(-183.868524764247,95.8895820176952,-3.32519803265031));
#29449=CARTESIAN_POINT('Ctrl Pts',(-184.640230357973,94.5993241361901,-2.59999275069374));
#29450=CARTESIAN_POINT('Ctrl Pts',(-184.295133716673,95.0116489254231,-3.26945356760231));
#29451=CARTESIAN_POINT('Ctrl Pts',(-184.188363389419,95.5840555999993,-3.90037822873724));
#29452=CARTESIAN_POINT('Ctrl Pts',(-184.78434203569,94.426893415286,-2.77839839816462));
#29453=CARTESIAN_POINT('Ctrl Pts',(-184.441552692558,94.8377263261817,-3.49555218419125));
#29454=CARTESIAN_POINT('Ctrl Pts',(-184.357297442187,95.4219062735372,-4.1680134022079));
#29455=CARTESIAN_POINT('Ctrl Pts',(-185.081686343193,94.0693232210915,-3.1143754936061));
#29456=CARTESIAN_POINT('Ctrl Pts',(-184.743586343125,94.4771334873336,-3.92236858029529));
#29457=CARTESIAN_POINT('Ctrl Pts',(-184.705925080379,95.0853544967748,-4.67202934040196));
#29458=CARTESIAN_POINT('Ctrl Pts',(-185.233416268676,93.8859970214969,-3.27026141835536));
#29459=CARTESIAN_POINT('Ctrl Pts',(-184.897720023963,94.2922334135553,-4.12090822859617));
#29460=CARTESIAN_POINT('Ctrl Pts',(-184.883856541663,94.9126597774132,-4.90588156360651));
#29461=CARTESIAN_POINT('Ctrl Pts',(-185.69467972387,93.3258217356729,-3.71184482224262));
#29462=CARTESIAN_POINT('Ctrl Pts',(-185.366864517595,93.7265360394383,-4.6855524165187));
#29463=CARTESIAN_POINT('Ctrl Pts',(-185.424878850264,94.3844962534327,-5.56832292611329));
#29464=CARTESIAN_POINT('Ctrl Pts',(-186.010146579491,92.9389319284735,-3.97193425575934));
#29465=CARTESIAN_POINT('Ctrl Pts',(-185.687350973287,93.3362230628123,-5.01951580728777));
#29466=CARTESIAN_POINT('Ctrl Pts',(-185.795033412765,94.0190928215223,-5.95849601722182));
#29467=CARTESIAN_POINT('Ctrl Pts',(-186.648836664447,92.1470885487441,-4.45009979324727));
#29468=CARTESIAN_POINT('Ctrl Pts',(-186.336019695174,92.5375609708031,-5.63706525171897));
#29469=CARTESIAN_POINT('Ctrl Pts',(-186.544745323736,93.2698431415528,-6.67581600087155));
#29470=CARTESIAN_POINT('Ctrl Pts',(-186.972201554671,91.741974605203,-4.66770157630044));
#29471=CARTESIAN_POINT('Ctrl Pts',(-186.664462004782,92.1288597295902,-5.91981377516862));
#29472=CARTESIAN_POINT('Ctrl Pts',(-186.924468369905,92.8858476278282,-7.00225129807417));
#29473=CARTESIAN_POINT('Ctrl Pts',(-187.622975925479,90.9175328418992,-5.07270906192872));
#29474=CARTESIAN_POINT('Ctrl Pts',(-187.325327673611,91.2972402661008,-6.44944820677759));
#29475=CARTESIAN_POINT('Ctrl Pts',(-187.688972154269,92.1029529048828,-7.60982332854755));
#29476=CARTESIAN_POINT('Ctrl Pts',(-187.951135111485,90.4972347714145,-5.26033203020097));
#29477=CARTESIAN_POINT('Ctrl Pts',(-187.658573120978,90.8732133787086,-6.69644438830181));
#29478=CARTESIAN_POINT('Ctrl Pts',(-188.074634250876,91.7031292223758,-7.89128595957309));
#29479=CARTESIAN_POINT('Ctrl Pts',(-188.605044860185,89.6501506723977,-5.61022454744543));
#29480=CARTESIAN_POINT('Ctrl Pts',(-188.322538615507,90.0186811388234,-7.16027924921534));
#29481=CARTESIAN_POINT('Ctrl Pts',(-188.843435098385,90.8958628411168,-8.41617737112857));
#29482=CARTESIAN_POINT('Ctrl Pts',(-188.930864921547,89.2233084878171,-5.77255548082708));
#29483=CARTESIAN_POINT('Ctrl Pts',(-188.653339852176,89.5880484625308,-7.37702489960499));
#29484=CARTESIAN_POINT('Ctrl Pts',(-189.226654411641,90.4883717460544,-8.65969820825197));
#29485=CARTESIAN_POINT('Ctrl Pts',(-189.903920178562,87.9339173140976,-6.23019362937991));
#29486=CARTESIAN_POINT('Ctrl Pts',(-189.64422831163,88.2832647934035,-7.99452678846992));
#29487=CARTESIAN_POINT('Ctrl Pts',(-190.371578955361,89.2552993716194,-9.34622475164829));
#29488=CARTESIAN_POINT('Ctrl Pts',(-190.546703712354,87.0625533618215,-6.49656692485956));
#29489=CARTESIAN_POINT('Ctrl Pts',(-190.296635791104,87.4039672654561,-8.35854013664169));
#29490=CARTESIAN_POINT('Ctrl Pts',(-191.128495190513,88.4191654814962,-9.74582492495691));
#29491=CARTESIAN_POINT('Ctrl Pts',(-191.817379516886,85.2993336154583,-6.97723500735076));
#29492=CARTESIAN_POINT('Ctrl Pts',(-191.58631881165,85.6248497292438,-9.02658828514773));
#29493=CARTESIAN_POINT('Ctrl Pts',(-192.625914150862,86.721646050191,-10.4669000807354));
#29494=CARTESIAN_POINT('Ctrl Pts',(-192.445310869352,84.4074358145282,-7.19119018591865));
#29495=CARTESIAN_POINT('Ctrl Pts',(-192.223411761402,84.7247818509418,-9.32938769806592));
#29496=CARTESIAN_POINT('Ctrl Pts',(-193.36646245408,85.8602217891397,-10.7878654563762));
#29497=CARTESIAN_POINT('Ctrl Pts',(-194.304305684022,81.7033032878079,-7.77457703832778));
#29498=CARTESIAN_POINT('Ctrl Pts',(-194.121426915844,81.9789046691737,-10.1764823230672));
#29499=CARTESIAN_POINT('Ctrl Pts',(-195.560439767958,83.2403639888807,-11.66303604594));
#29500=CARTESIAN_POINT('Ctrl Pts',(-195.510473766748,79.8627399618138,-8.08647138287587));
#29501=CARTESIAN_POINT('Ctrl Pts',(-195.343662380556,80.1208834365032,-10.6467860035186));
#29502=CARTESIAN_POINT('Ctrl Pts',(-196.986083554655,81.4464501527923,-12.1309258408888));
#29503=CARTESIAN_POINT('Ctrl Pts',(-197.26422362369,77.0498973143794,-8.48148993785693));
#29504=CARTESIAN_POINT('Ctrl Pts',(-197.110469889354,77.3001806896492,-11.2686726614448));
#29505=CARTESIAN_POINT('Ctrl Pts',(-199.061639908547,78.6896512667519,-12.7235158739264));
#29506=CARTESIAN_POINT('Ctrl Pts',(-197.839595055258,76.1035745652819,-8.60067013564272));
#29507=CARTESIAN_POINT('Ctrl Pts',(-197.693451452524,76.3452591128515,-11.4629048769373));
#29508=CARTESIAN_POINT('Ctrl Pts',(-199.743053232215,77.7596906841316,-12.9023052799916));
#29509=CARTESIAN_POINT('Ctrl Pts',(-198.971269927631,74.1939245965756,-8.81827543079709));
#29510=CARTESIAN_POINT('Ctrl Pts',(-198.840144887273,74.4184120242095,-11.8283305042784));
#29511=CARTESIAN_POINT('Ctrl Pts',(-201.084141185834,75.8782216647446,-13.2287486186965));
#29512=CARTESIAN_POINT('Ctrl Pts',(-199.528026213893,73.2297480452024,-8.9167473697722));
#29513=CARTESIAN_POINT('Ctrl Pts',(-199.403933368659,73.4456397089867,-11.999284368886));
#29514=CARTESIAN_POINT('Ctrl Pts',(-201.744353740694,74.9258683491321,-13.3764727664485));
#29515=CARTESIAN_POINT('Ctrl Pts',(-201.161792437304,70.3249942677904,-9.18473475784064));
#29516=CARTESIAN_POINT('Ctrl Pts',(-201.069113535252,70.4962985183013,-12.4841466691128));
#29517=CARTESIAN_POINT('Ctrl Pts',(-203.682864677576,72.0498212174151,-13.7784991672417));
#29518=CARTESIAN_POINT('Ctrl Pts',(-202.204497602129,68.3686954361411,-9.327550429722));
#29519=CARTESIAN_POINT('Ctrl Pts',(-202.122699464231,68.5235270163752,-12.7632527718059));
#29520=CARTESIAN_POINT('Ctrl Pts',(-204.921631000465,70.1037195380372,-13.9927475603924));
#29521=CARTESIAN_POINT('Ctrl Pts',(-204.197844600951,64.4174374747376,-9.56200891039826));
#29522=CARTESIAN_POINT('Ctrl Pts',(-204.139132956947,64.5385208888658,-13.2647553306726));
#29523=CARTESIAN_POINT('Ctrl Pts',(-207.292248848856,66.1565464226095,-14.3444784427628));
#29524=CARTESIAN_POINT('Ctrl Pts',(-205.148489282526,62.4224747699383,-9.6535097636974));
#29525=CARTESIAN_POINT('Ctrl Pts',(-205.098222238211,62.5281076726303,-13.4851030107949));
#29526=CARTESIAN_POINT('Ctrl Pts',(-208.424103723681,64.1554710849893,-14.4817477042882));
#29527=CARTESIAN_POINT('Ctrl Pts',(-207.863010265155,56.3804553729788,-9.87162265399631));
#29528=CARTESIAN_POINT('Ctrl Pts',(-207.874530509962,56.3622740214675,-14.0896831956044));
#29529=CARTESIAN_POINT('Ctrl Pts',(-211.659039648998,58.0728675461335,-14.8089642189829));
#29530=CARTESIAN_POINT('Ctrl Pts',(-209.489746376511,52.2763554538315,-9.94272550904972));
#29531=CARTESIAN_POINT('Ctrl Pts',(-209.500567148536,52.239261066085,-14.3961534366159));
#29532=CARTESIAN_POINT('Ctrl Pts',(-213.601767269327,53.9120928346637,-14.9156391942734));
#29533=CARTESIAN_POINT('Ctrl Pts',(-211.653837598457,46.0069427729526,-9.99217179438664));
#29534=CARTESIAN_POINT('Ctrl Pts',(-211.654748063316,46.0028378682449,-14.7791601532076));
#29535=CARTESIAN_POINT('Ctrl Pts',(-216.189589140866,47.5215622113001,-14.9898323220643));
#29536=CARTESIAN_POINT('Ctrl Pts',(-212.329136320276,43.8982352536057,-9.99883253041345));
#29537=CARTESIAN_POINT('Ctrl Pts',(-212.331887292226,43.8852959564764,-14.8942914798601));
#29538=CARTESIAN_POINT('Ctrl Pts',(-216.99775401071,45.3664543056449,-14.99982994474));
#29539=CARTESIAN_POINT('Ctrl Pts',(-213.586563915695,39.6427642163839,-9.99904901899915));
#29540=CARTESIAN_POINT('Ctrl Pts',(-213.594819890769,39.6109883608531,-15.1032774268557));
#29541=CARTESIAN_POINT('Ctrl Pts',(-218.503477700196,41.0074627753361,-15.0001657416214));
#29542=CARTESIAN_POINT('Ctrl Pts',(-214.169149505489,37.4941453785589,-9.99258591104121));
#29543=CARTESIAN_POINT('Ctrl Pts',(-214.177547647221,37.4569157620953,-15.1964629582924));
#29544=CARTESIAN_POINT('Ctrl Pts',(-219.201583812779,38.8016704170055,-14.99047558146));
#29545=CARTESIAN_POINT('Ctrl Pts',(-215.771854048122,31.0022455423769,-9.96182684240677));
#29546=CARTESIAN_POINT('Ctrl Pts',(-215.799160452695,30.8835450730081,-15.4509064845787));
#29547=CARTESIAN_POINT('Ctrl Pts',(-221.123034242247,32.1244801171726,-14.9443482381631));
#29548=CARTESIAN_POINT('Ctrl Pts',(-216.636779994235,26.656889293641,-9.92696752601132));
#29549=CARTESIAN_POINT('Ctrl Pts',(-216.651517550254,26.5601579572741,-15.5778765399567));
#29550=CARTESIAN_POINT('Ctrl Pts',(-222.161298573218,27.6385960407911,-14.8920638015871));
#29551=CARTESIAN_POINT('Ctrl Pts',(-217.971708585098,17.9323050948719,-9.86264007720543));
#29552=CARTESIAN_POINT('Ctrl Pts',(-217.98395218067,17.8351858692922,-15.7751687151717));
#29553=CARTESIAN_POINT('Ctrl Pts',(-223.764494274026,18.6116604334835,-14.7955788665586));
#29554=CARTESIAN_POINT('Ctrl Pts',(-218.441684997606,13.5530627335445,-9.83311016810406));
#29555=CARTESIAN_POINT('Ctrl Pts',(-218.444591836418,13.4953035845419,-15.8420879379444));
#29556=CARTESIAN_POINT('Ctrl Pts',(-224.3293991122,14.0705718828394,-14.7512857241696));
#29557=CARTESIAN_POINT('Ctrl Pts',(-218.98892491974,4.76083842406514,-9.79797621148514));
#29558=CARTESIAN_POINT('Ctrl Pts',(-218.989185405442,4.72249428361865,-15.9213704338492));
#29559=CARTESIAN_POINT('Ctrl Pts',(-224.987222679375,4.94518643901801,-14.6985866952544));
#29560=CARTESIAN_POINT('Ctrl Pts',(-219.066199483219,0.347844039587536,
-9.79239498047612));
#29561=CARTESIAN_POINT('Ctrl Pts',(-219.064738571508,0.358452420802183,
-15.9323153280885));
#29562=CARTESIAN_POINT('Ctrl Pts',(-225.08015488072,0.360857152534145,-14.6902150849217));
#29563=CARTESIAN_POINT('Ctrl Pts',(-218.882089664708,-6.29742822354361,
-9.80469739981719));
#29564=CARTESIAN_POINT('Ctrl Pts',(-218.881384487388,-6.27783716390587,
-15.9056638247615));
#29565=CARTESIAN_POINT('Ctrl Pts',(-224.858807959456,-6.53966795784784,
-14.7086681091492));
#29566=CARTESIAN_POINT('Ctrl Pts',(-218.770640597971,-8.5168252216966,-9.81212408241458));
#29567=CARTESIAN_POINT('Ctrl Pts',(-218.77099042416,-8.48718110804912,-15.8896189712452));
#29568=CARTESIAN_POINT('Ctrl Pts',(-224.724819198552,-8.84385385870031,
-14.7198077601516));
#29569=CARTESIAN_POINT('Ctrl Pts',(-218.445706585932,-12.9643846257828,
-9.83258697597486));
#29570=CARTESIAN_POINT('Ctrl Pts',(-218.447558735051,-12.9256116392978,
-15.8424934042915));
#29571=CARTESIAN_POINT('Ctrl Pts',(-224.334251471307,-13.4588585853863,
-14.7505009402079));
#29572=CARTESIAN_POINT('Ctrl Pts',(-218.233279978387,-15.1775360624383,
-9.84554950482581));
#29573=CARTESIAN_POINT('Ctrl Pts',(-218.236862025186,-15.1309441945871,
-15.8117609314217));
#29574=CARTESIAN_POINT('Ctrl Pts',(-224.078945146157,-15.754094702541,-14.769943939359));
#29575=CARTESIAN_POINT('Ctrl Pts',(-217.44965178097,-21.7782118624344,-9.88922208942823));
#29576=CARTESIAN_POINT('Ctrl Pts',(-217.459829407993,-21.6907915561905,
-15.6977966994989));
#29577=CARTESIAN_POINT('Ctrl Pts',(-223.13742499135,-22.5936734469255,-14.8354495694809));
#29578=CARTESIAN_POINT('Ctrl Pts',(-216.732153346241,-26.1303721630048,
-9.92513272450046));
#29579=CARTESIAN_POINT('Ctrl Pts',(-216.753951919438,-26.0158068183044,
-15.5940689166965));
#29580=CARTESIAN_POINT('Ctrl Pts',(-222.275639117307,-27.0954312018765,
-14.8893122662313));
#29581=CARTESIAN_POINT('Ctrl Pts',(-214.915312965014,-34.7401291355706,
-9.98260167196437));
#29582=CARTESIAN_POINT('Ctrl Pts',(-214.935762892442,-34.6425169654146,
-15.3168242444749));
#29583=CARTESIAN_POINT('Ctrl Pts',(-220.095831592936,-35.9737986453296,
-14.975504791654));
#29584=CARTESIAN_POINT('Ctrl Pts',(-213.815951507118,-38.997732367201,-10.0042638421583));
#29585=CARTESIAN_POINT('Ctrl Pts',(-213.847033440636,-38.893318416415,-15.1477002122303));
#29586=CARTESIAN_POINT('Ctrl Pts',(-218.777784106532,-40.3504347492802,
-15.0079905031581));
#29587=CARTESIAN_POINT('Ctrl Pts',(-211.234344254847,-47.4180803462803,
-9.99138542271174));
#29588=CARTESIAN_POINT('Ctrl Pts',(-211.252009920408,-47.3564561926427,
-14.7119977239021));
#29589=CARTESIAN_POINT('Ctrl Pts',(-215.687315361276,-48.9667036279376,
-14.9886489895387));
#29590=CARTESIAN_POINT('Ctrl Pts',(-209.75211504862,-51.5808392384507,-9.95731237985128));
#29591=CARTESIAN_POINT('Ctrl Pts',(-209.774784444065,-51.529992979264,-14.4524533619249));
#29592=CARTESIAN_POINT('Ctrl Pts',(-213.914906046157,-53.206374129089,-14.9375236211255));
#29593=CARTESIAN_POINT('Ctrl Pts',(-207.233810470461,-57.7518422440691,
-9.8166773227685));
#29594=CARTESIAN_POINT('Ctrl Pts',(-207.20309976548,-57.8216061018363,-13.9396592655048));
#29595=CARTESIAN_POINT('Ctrl Pts',(-210.909503771198,-59.4516238932021,
-14.7265343478991));
#29596=CARTESIAN_POINT('Ctrl Pts',(-206.343367468842,-59.8001282170186,
-9.75447731805782));
#29597=CARTESIAN_POINT('Ctrl Pts',(-206.306005665109,-59.8842764834739,
-13.7521834792451));
#29598=CARTESIAN_POINT('Ctrl Pts',(-209.847720713297,-61.5177848329008,
-14.6332201986806));
#29599=CARTESIAN_POINT('Ctrl Pts',(-204.476765026371,-63.8405295173718,
-9.58938895529315));
#29600=CARTESIAN_POINT('Ctrl Pts',(-204.419864648177,-63.9571626937035,
-13.329314053494));
#29601=CARTESIAN_POINT('Ctrl Pts',(-207.624289029391,-65.5783610758614,
-14.3855537798929));
#29602=CARTESIAN_POINT('Ctrl Pts',(-203.49960767437,-65.8355428611045,-9.48655973173275));
#29603=CARTESIAN_POINT('Ctrl Pts',(-203.433512500785,-65.968284694467,-13.0953532628466));
#29604=CARTESIAN_POINT('Ctrl Pts',(-206.461446708194,-67.5757325777054,
-14.2312904187871));
#29605=CARTESIAN_POINT('Ctrl Pts',(-201.45887205873,-69.7747638156398,-9.22591935843988));
#29606=CARTESIAN_POINT('Ctrl Pts',(-201.368484720857,-69.941659180332,-12.5633651459106));
#29607=CARTESIAN_POINT('Ctrl Pts',(-204.03575029879,-71.5029679315967,-13.8402831180884));
#29608=CARTESIAN_POINT('Ctrl Pts',(-200.395284333713,-71.7189792947419,
-9.06826475769951));
#29609=CARTESIAN_POINT('Ctrl Pts',(-200.2932655858,-71.90279735052,-12.2674645147884));
#29610=CARTESIAN_POINT('Ctrl Pts',(-202.772885289101,-73.432839265888,-13.6037743174855));
#29611=CARTESIAN_POINT('Ctrl Pts',(-198.18283411717,-75.5555694788219,-8.67680237261049));
#29612=CARTESIAN_POINT('Ctrl Pts',(-198.051808705163,-75.7741525073902,
-11.5869496831444));
#29613=CARTESIAN_POINT('Ctrl Pts',(-200.149286733965,-77.222776724018,-13.0165160576299));
#29614=CARTESIAN_POINT('Ctrl Pts',(-197.033949531596,-77.4479653439144,
-8.44340981108465));
#29615=CARTESIAN_POINT('Ctrl Pts',(-196.888887581277,-77.6837498187098,
-11.205475577738));
#29616=CARTESIAN_POINT('Ctrl Pts',(-198.788527494164,-79.0828624701376,
-12.6663899188091));
#29617=CARTESIAN_POINT('Ctrl Pts',(-195.247729756749,-80.2461536453752,
-8.00941135562084));
#29618=CARTESIAN_POINT('Ctrl Pts',(-195.066101080631,-80.5254857528079,
-10.530388667617));
#29619=CARTESIAN_POINT('Ctrl Pts',(-196.6758925451,-81.8181682371439,-12.0153234692363));
#29620=CARTESIAN_POINT('Ctrl Pts',(-194.6416840559,-81.1723200972973,-7.85053644481165));
#29621=CARTESIAN_POINT('Ctrl Pts',(-194.451609817737,-81.4601421251086,
-10.2906945195429));
#29622=CARTESIAN_POINT('Ctrl Pts',(-195.959582481097,-82.7209577867424,
-11.7769863872961));
#29623=CARTESIAN_POINT('Ctrl Pts',(-193.414428959512,-83.0027585457057,
-7.49863868716929));
#29624=CARTESIAN_POINT('Ctrl Pts',(-193.206673895877,-83.3072532983952,
-9.77173373334771));
#29625=CARTESIAN_POINT('Ctrl Pts',(-194.510093498015,-84.4999373718914,
-11.2490853481395));
#29626=CARTESIAN_POINT('Ctrl Pts',(-192.792617590937,-83.9079862550153,
-7.30555612066123));
#29627=CARTESIAN_POINT('Ctrl Pts',(-192.575907971764,-84.2208076263337,
-9.49288654034082));
#29628=CARTESIAN_POINT('Ctrl Pts',(-193.776202443296,-85.3770629978107,
-10.9594318944836));
#29629=CARTESIAN_POINT('Ctrl Pts',(-191.534262284156,-85.6970547926546,
-6.87464494826575));
#29630=CARTESIAN_POINT('Ctrl Pts',(-191.298951356079,-86.0260858611082,
-8.8826451632366));
#29631=CARTESIAN_POINT('Ctrl Pts',(-192.292150323284,-87.1051898982516,
-10.3129993370047));
#29632=CARTESIAN_POINT('Ctrl Pts',(-190.897692592206,-86.5809228644259,
-6.63700227874789));
#29633=CARTESIAN_POINT('Ctrl Pts',(-190.652958604134,-86.9180526562817,
-8.55216637333298));
#29634=CARTESIAN_POINT('Ctrl Pts',(-191.541959253817,-87.9562162178622,
-9.95649928586201));
#29635=CARTESIAN_POINT('Ctrl Pts',(-189.584682347239,-88.3624698219694,
-6.08799905112524));
#29636=CARTESIAN_POINT('Ctrl Pts',(-189.320453977114,-88.7150993305577,
-7.80170139306956));
#29637=CARTESIAN_POINT('Ctrl Pts',(-189.995794337287,-89.6659208608691,
-9.13291138381351));
#29638=CARTESIAN_POINT('Ctrl Pts',(-188.907584299326,-89.2592395987802,
-5.77452884411308));
#29639=CARTESIAN_POINT('Ctrl Pts',(-188.633022709524,-89.6201125002178,
-7.38005660091507));
#29640=CARTESIAN_POINT('Ctrl Pts',(-189.199000170436,-90.5235796561882,
-8.66259199213005));
#29641=CARTESIAN_POINT('Ctrl Pts',(-188.226751608154,-90.1401577923431,
-5.4077170003843));
#29642=CARTESIAN_POINT('Ctrl Pts',(-187.93744048601,-90.5142672861031,-6.89114911006534));
#29643=CARTESIAN_POINT('Ctrl Pts',(-188.39869005518,-91.362817758299,-8.1123941340948));
#29644=CARTESIAN_POINT('Origin',(-71.5953323638214,6.93889390390723E-15,
-26.5));
#29645=CARTESIAN_POINT('Ctrl Pts',(-188.850942384682,90.9673968784446,5.31766757924555));
#29646=CARTESIAN_POINT('Ctrl Pts',(-189.341118335966,90.3355674301194,5.58646961538285));
#29647=CARTESIAN_POINT('Ctrl Pts',(-189.830924097054,89.6936385792413,5.82722845321623));
#29648=CARTESIAN_POINT('Ctrl Pts',(-190.318786696358,89.0431674195335,6.04773461915937));
#29649=CARTESIAN_POINT('Ctrl Pts',(-190.482667264906,88.8246641285877,6.1218060398724));
#29650=CARTESIAN_POINT('Ctrl Pts',(-190.646328518149,88.6051970380796,6.19359259998661));
#29651=CARTESIAN_POINT('Ctrl Pts',(-190.809710697124,88.3848254779465,6.2633908242173));
#29652=CARTESIAN_POINT('Ctrl Pts',(-190.810466894386,88.3838055113162,6.26371387797037));
#29653=CARTESIAN_POINT('Ctrl Pts',(-190.811223085654,88.3827855253331,6.26403688911534));
#29654=CARTESIAN_POINT('Ctrl Pts',(-190.81197927092,88.3817655200031,6.26435985768164));
#29655=CARTESIAN_POINT('Ctrl Pts',(-191.415025663252,87.5683265894712,6.5219224384322));
#29656=CARTESIAN_POINT('Ctrl Pts',(-192.014372732003,86.7424513122927,6.75185269721188));
#29657=CARTESIAN_POINT('Ctrl Pts',(-192.608472917412,85.9055593357088,6.96149402186932));
#29658=CARTESIAN_POINT('Ctrl Pts',(-192.653739491705,85.8417936043329,6.97746732878041));
#29659=CARTESIAN_POINT('Ctrl Pts',(-192.698975604839,85.7779639226609,6.99332287300553));
#29660=CARTESIAN_POINT('Ctrl Pts',(-192.74418057204,85.7140709218425,7.00906391406534));
#29661=CARTESIAN_POINT('Ctrl Pts',(-192.745135383982,85.7127213843022,7.00939639376675));
#29662=CARTESIAN_POINT('Ctrl Pts',(-192.746090182109,85.7113718184013,7.00972882239919));
#29663=CARTESIAN_POINT('Ctrl Pts',(-192.747044966413,85.7100222241461,7.01006119999323));
#29664=CARTESIAN_POINT('Ctrl Pts',(-193.340906354287,84.8705950215575,7.21679503344427));
#29665=CARTESIAN_POINT('Ctrl Pts',(-193.930245240205,84.0189651457988,7.40382485455509));
#29666=CARTESIAN_POINT('Ctrl Pts',(-194.511008670157,83.1605775933826,7.57462063256265));
#29667=CARTESIAN_POINT('Ctrl Pts',(-194.554435141729,83.0963918325032,7.58739185336559));
#29668=CARTESIAN_POINT('Ctrl Pts',(-194.597813668124,83.0321683003785,7.60007232470945));
#29669=CARTESIAN_POINT('Ctrl Pts',(-194.641142556604,82.9679092789718,7.61266350630674));
#29670=CARTESIAN_POINT('Ctrl Pts',(-194.64192321951,82.9667515148069,7.61289036346279));
#29671=CARTESIAN_POINT('Ctrl Pts',(-194.642703866312,82.9655937391075,7.61311719163327));
#29672=CARTESIAN_POINT('Ctrl Pts',(-194.643484497,82.9644359518865,7.6133439908268));
#29673=CARTESIAN_POINT('Ctrl Pts',(-195.26639704584,82.0405673424527,7.79432081605224));
#29674=CARTESIAN_POINT('Ctrl Pts',(-195.879202354609,81.109240118497,7.95688686492277));
#29675=CARTESIAN_POINT('Ctrl Pts',(-196.481682775292,80.1707231918713,8.10499840407016));
#29676=CARTESIAN_POINT('Ctrl Pts',(-196.482156857174,80.1699846884177,8.10511495059168));
#29677=CARTESIAN_POINT('Ctrl Pts',(-196.482630932664,80.1692461805125,8.10523148816305));
#29678=CARTESIAN_POINT('Ctrl Pts',(-196.48310500176,80.1685076681557,8.10534801678623));
#29679=CARTESIAN_POINT('Ctrl Pts',(-197.688784784991,78.2902805809609,8.40171031118339));
#29680=CARTESIAN_POINT('Ctrl Pts',(-198.853091809375,76.3833019518293,8.64076529068621));
#29681=CARTESIAN_POINT('Ctrl Pts',(-199.974927008656,74.4488082848391,8.84133536347261));
#29682=CARTESIAN_POINT('Ctrl Pts',(-199.975191724801,74.4483518080694,8.8413826914016));
#29683=CARTESIAN_POINT('Ctrl Pts',(-199.975456438584,74.4478953297663,8.84143001716346));
#29684=CARTESIAN_POINT('Ctrl Pts',(-199.975721150003,74.4474388499298,8.84147734075833));
#29685=CARTESIAN_POINT('Ctrl Pts',(-201.097094425615,72.5136942047661,9.04195004698192));
#29686=CARTESIAN_POINT('Ctrl Pts',(-202.176057085258,70.5524290707013,9.2035344356386));
#29687=CARTESIAN_POINT('Ctrl Pts',(-203.211775255623,68.564256990898,9.33720992260623));
#29688=CARTESIAN_POINT('Ctrl Pts',(-203.212835287712,68.5622221456433,9.33734673618142));
#29689=CARTESIAN_POINT('Ctrl Pts',(-203.213895274515,68.5601872721942,9.33748352035168));
#29690=CARTESIAN_POINT('Ctrl Pts',(-203.21495521603,68.5581523705511,9.33762027512486));
#29691=CARTESIAN_POINT('Ctrl Pts',(-204.249652408617,66.5717153948246,9.47111799919037));
#29692=CARTESIAN_POINT('Ctrl Pts',(-205.241200921077,64.5583939991535,9.57660331773388));
#29693=CARTESIAN_POINT('Ctrl Pts',(-206.188735439408,62.5184870637267,9.66139767362455));
#29694=CARTESIAN_POINT('Ctrl Pts',(-206.19056002032,62.5145590007537,9.66156095439187));
#29695=CARTESIAN_POINT('Ctrl Pts',(-206.192384445048,62.5106308228101,9.66172415830768));
#29696=CARTESIAN_POINT('Ctrl Pts',(-206.194208713484,62.5067025301279,9.66188728540609));
#29697=CARTESIAN_POINT('Ctrl Pts',(-206.666525419703,61.4896382516984,9.7041221080299));
#29698=CARTESIAN_POINT('Ctrl Pts',(-207.128379381789,60.4648516858952,9.74120877012034));
#29699=CARTESIAN_POINT('Ctrl Pts',(-207.577897027375,59.4364154683561,9.77373815047265));
#29700=CARTESIAN_POINT('Ctrl Pts',(-207.580068445556,59.431447554144,9.77389528532283));
#29701=CARTESIAN_POINT('Ctrl Pts',(-207.582239572049,59.4264795655298,9.77405231379252));
#29702=CARTESIAN_POINT('Ctrl Pts',(-207.584410406868,59.4215115025229,9.77420923596013));
#29703=CARTESIAN_POINT('Ctrl Pts',(-208.033367357209,58.3940512842233,9.80666278664411));
#29704=CARTESIAN_POINT('Ctrl Pts',(-208.469851754248,57.3634026279674,9.83457096111565));
#29705=CARTESIAN_POINT('Ctrl Pts',(-208.893990826528,56.3295993288226,9.85862681314411));
#29706=CARTESIAN_POINT('Ctrl Pts',(-208.896457271165,56.3235875775624,9.85876670223024));
#29707=CARTESIAN_POINT('Ctrl Pts',(-208.898923299152,56.3175757198386,9.8589064637187));
#29708=CARTESIAN_POINT('Ctrl Pts',(-208.901388910506,56.3115637556553,9.85904609770791));
#29709=CARTESIAN_POINT('Ctrl Pts',(-210.603104765652,52.1622258018391,9.95541869631808));
#29710=CARTESIAN_POINT('Ctrl Pts',(-212.106358542097,47.9621739982348,9.99108073365087));
#29711=CARTESIAN_POINT('Ctrl Pts',(-213.416141475183,43.7127381801167,9.99852944383294));
#29712=CARTESIAN_POINT('Ctrl Pts',(-213.419320039466,43.7024257042292,9.99854752026648));
#29713=CARTESIAN_POINT('Ctrl Pts',(-213.422497464223,43.6921129374695,9.99856542770493));
#29714=CARTESIAN_POINT('Ctrl Pts',(-213.425673749455,43.6817998798392,9.99858316645284));
#29715=CARTESIAN_POINT('Ctrl Pts',(-214.733236103275,39.4362850960293,10.0058855707623));
#29716=CARTESIAN_POINT('Ctrl Pts',(-215.847686530337,35.1414767092267,9.98461098471693));
#29717=CARTESIAN_POINT('Ctrl Pts',(-216.769233470622,30.7974644027352,9.95600465872816));
#29718=CARTESIAN_POINT('Ctrl Pts',(-216.772375208496,30.7826547957672,9.9559071340402));
#29719=CARTESIAN_POINT('Ctrl Pts',(-216.775514704529,30.7678446169708,9.95580952290657));
#29720=CARTESIAN_POINT('Ctrl Pts',(-216.778651958541,30.7530338663012,9.95571182588763));
#29721=CARTESIAN_POINT('Ctrl Pts',(-217.69798150674,26.4129451558353,9.92708304545502));
#29722=CARTESIAN_POINT('Ctrl Pts',(-218.424787910683,22.0237499448137,9.89108693511256));
#29723=CARTESIAN_POINT('Ctrl Pts',(-218.954543661828,17.5843174969628,9.86183278666612));
#29724=CARTESIAN_POINT('Ctrl Pts',(-218.956871344149,17.5648111708836,9.86170424749687));
#29725=CARTESIAN_POINT('Ctrl Pts',(-218.959195214687,17.5453038729898,9.86157582861175));
#29726=CARTESIAN_POINT('Ctrl Pts',(-218.961515272787,17.5257956031157,9.86144753085713));
#29727=CARTESIAN_POINT('Ctrl Pts',(-219.091650787911,16.4315476833897,9.85425111866854));
#29728=CARTESIAN_POINT('Ctrl Pts',(-219.209795922764,15.3341948244095,9.84743578264517));
#29729=CARTESIAN_POINT('Ctrl Pts',(-219.31582170744,14.2338471358419,9.84115131033219));
#29730=CARTESIAN_POINT('Ctrl Pts',(-219.317817511001,14.2131344588084,9.84103301295519));
#29731=CARTESIAN_POINT('Ctrl Pts',(-219.31980905213,14.192420238668,9.84091490168962));
#29732=CARTESIAN_POINT('Ctrl Pts',(-219.321796327431,14.1717045123362,9.84079697751308));
#29733=CARTESIAN_POINT('Ctrl Pts',(-219.427264023453,13.0722896869807,9.83453856369359));
#29734=CARTESIAN_POINT('Ctrl Pts',(-219.520734074763,11.9684395739338,9.82880673133093));
#29735=CARTESIAN_POINT('Ctrl Pts',(-219.601691870632,10.8656763132971,9.82374740145546));
#29736=CARTESIAN_POINT('Ctrl Pts',(-219.603297940124,10.8437993042859,9.82364703267349));
#29737=CARTESIAN_POINT('Ctrl Pts',(-219.604899106509,10.8219226927283,9.82354693073774));
#29738=CARTESIAN_POINT('Ctrl Pts',(-219.606495370559,10.8000464796908,9.82344709613719));
#29739=CARTESIAN_POINT('Ctrl Pts',(-219.768858415878,8.5749205235309,9.81329247931069));
#29740=CARTESIAN_POINT('Ctrl Pts',(-219.880517558162,6.35371483186536,9.80590845216625));
#29741=CARTESIAN_POINT('Ctrl Pts',(-219.942344006131,4.13636470843061,9.80180544072015));
#29742=CARTESIAN_POINT('Ctrl Pts',(-219.943012881674,4.11237608680465,9.801761051885));
#29743=CARTESIAN_POINT('Ctrl Pts',(-219.943675933535,4.08838791580208,9.8017170610927));
#29744=CARTESIAN_POINT('Ctrl Pts',(-219.944333162218,4.06440019538434,9.80167346805754));
#29745=CARTESIAN_POINT('Ctrl Pts',(-220.066370321029,-0.389746924528067,
9.79357891848717));
#29746=CARTESIAN_POINT('Ctrl Pts',(-219.987631786347,-4.82836129360515,
9.79922661021772));
#29747=CARTESIAN_POINT('Ctrl Pts',(-219.711339275957,-9.25169566130756,
9.81683113342425));
#29748=CARTESIAN_POINT('Ctrl Pts',(-219.709579972076,-9.27986142413934,
9.81694323094711));
#29749=CARTESIAN_POINT('Ctrl Pts',(-219.707812658021,-9.30802656742054,
9.81705581248959));
#29750=CARTESIAN_POINT('Ctrl Pts',(-219.706037333374,-9.3361910911259,9.81716887563367));
#29751=CARTESIAN_POINT('Ctrl Pts',(-219.427502399894,-13.7549906314892,
9.83490762294272));
#29752=CARTESIAN_POINT('Ctrl Pts',(-218.951784949751,-18.1585397204247,
9.86451878801393));
#29753=CARTESIAN_POINT('Ctrl Pts',(-218.277266277532,-22.5467434353284,
9.89667505290868));
#29754=CARTESIAN_POINT('Ctrl Pts',(-218.272304508842,-22.579023122596,9.89691159483835));
#29755=CARTESIAN_POINT('Ctrl Pts',(-218.267331966596,-22.6113019783348,
9.89714824949614));
#29756=CARTESIAN_POINT('Ctrl Pts',(-218.262348648669,-22.6435800023996,
9.8973850108931));
#29757=CARTESIAN_POINT('Ctrl Pts',(-217.926448866683,-24.8192752731317,
9.91334387661025));
#29758=CARTESIAN_POINT('Ctrl Pts',(-217.541590744706,-26.9911917525532,
9.92978970018313));
#29759=CARTESIAN_POINT('Ctrl Pts',(-217.107123822393,-29.1592853602726,
9.94488796227917));
#29760=CARTESIAN_POINT('Ctrl Pts',(-217.100247949909,-29.1935976045774,
9.94512690733937));
#29761=CARTESIAN_POINT('Ctrl Pts',(-217.093359647348,-29.2279088910387,
9.94536550728949));
#29762=CARTESIAN_POINT('Ctrl Pts',(-217.086458911175,-29.2622192194123,
9.94560375335194));
#29763=CARTESIAN_POINT('Ctrl Pts',(-216.872106429072,-30.3279756639031,
9.95300421520923));
#29764=CARTESIAN_POINT('Ctrl Pts',(-216.645741368245,-31.3928784273454,
9.96006389214994));
#29765=CARTESIAN_POINT('Ctrl Pts',(-216.407304521944,-32.4567111069465,
9.96651848904424));
#29766=CARTESIAN_POINT('Ctrl Pts',(-216.399387998386,-32.4920322269846,
9.96673279303779));
#29767=CARTESIAN_POINT('Ctrl Pts',(-216.391457819029,-32.5273535271178,
9.96694643567054));
#29768=CARTESIAN_POINT('Ctrl Pts',(-216.383514027764,-32.5626748172608,
9.96715940532502));
#29769=CARTESIAN_POINT('Ctrl Pts',(-216.144496659423,-33.6254421451658,
9.97356735898984));
#29770=CARTESIAN_POINT('Ctrl Pts',(-215.893087346094,-34.6884985009459,
9.9793701644089));
#29771=CARTESIAN_POINT('Ctrl Pts',(-215.630475785694,-35.7466478938294,
9.98424576551855));
#29772=CARTESIAN_POINT('Ctrl Pts',(-215.621483320461,-35.7828815295937,
9.98441271808302));
#29773=CARTESIAN_POINT('Ctrl Pts',(-215.612477740882,-35.8191096434725,
9.98457862995805));
#29774=CARTESIAN_POINT('Ctrl Pts',(-215.603459052608,-35.8553322274098,
9.98474348708846));
#29775=CARTESIAN_POINT('Ctrl Pts',(-214.523945905845,-40.19107977512,10.0044764498213));
#29776=CARTESIAN_POINT('Ctrl Pts',(-213.25628871331,-44.4489165154168,10.0091772927501));
#29777=CARTESIAN_POINT('Ctrl Pts',(-211.806023480029,-48.6303143412221,
9.97506610014392));
#29778=CARTESIAN_POINT('Ctrl Pts',(-211.792493566962,-48.6693237222522,
9.97474786768549));
#29779=CARTESIAN_POINT('Ctrl Pts',(-211.778947757168,-48.708326450718,9.9744263118785));
#29780=CARTESIAN_POINT('Ctrl Pts',(-211.765386051776,-48.7473225261173,
9.97410140367428));
#29781=CARTESIAN_POINT('Ctrl Pts',(-210.3130864592,-52.9233448463522,9.93930754560066));
#29782=CARTESIAN_POINT('Ctrl Pts',(-208.67849395231,-57.0230760419839,9.86612985349125));
#29783=CARTESIAN_POINT('Ctrl Pts',(-206.863010141496,-61.0458903190202,
9.71890425900672));
#29784=CARTESIAN_POINT('Ctrl Pts',(-206.844340078596,-61.0872601154014,
9.71739022120968));
#29785=CARTESIAN_POINT('Ctrl Pts',(-206.825650859292,-61.1286217636414,
9.71586826024716));
#29786=CARTESIAN_POINT('Ctrl Pts',(-206.80694248212,-61.1699752611634,9.71433831653629));
#29787=CARTESIAN_POINT('Ctrl Pts',(-205.90751707084,-63.1580892582013,9.64078462244658));
#29788=CARTESIAN_POINT('Ctrl Pts',(-204.963811205864,-65.1273654886791,
9.54879048714052));
#29789=CARTESIAN_POINT('Ctrl Pts',(-203.975665504039,-67.0775131761083,
9.43173502720273));
#29790=CARTESIAN_POINT('Ctrl Pts',(-202.966926805213,-69.0683020214223,
9.31224012667321));
#29791=CARTESIAN_POINT('Ctrl Pts',(-201.911874129873,-71.0391603800216,
9.16677547320627));
#29792=CARTESIAN_POINT('Ctrl Pts',(-200.810136447587,-72.9895868038661,
8.98489141523638));
#29793=CARTESIAN_POINT('Ctrl Pts',(-200.785750305287,-73.0327580388001,
8.98086554719985));
#29794=CARTESIAN_POINT('Ctrl Pts',(-200.761341285003,-73.0759192572446,
8.97682171266042));
#29795=CARTESIAN_POINT('Ctrl Pts',(-200.73690938147,-73.1190704516511,8.97275974828342));
#29796=CARTESIAN_POINT('Ctrl Pts',(-200.209418061294,-74.0507162595116,
8.88506085290961));
#29797=CARTESIAN_POINT('Ctrl Pts',(-199.671247876679,-74.9777097146329,
8.78891298975294));
#29798=CARTESIAN_POINT('Ctrl Pts',(-199.122382643862,-75.899913195448,8.68267567009917));
#29799=CARTESIAN_POINT('Ctrl Pts',(-199.09648849205,-75.9434205548256,8.67766364689428));
#29800=CARTESIAN_POINT('Ctrl Pts',(-199.070569960254,-75.9869180195701,
8.67262900795918));
#29801=CARTESIAN_POINT('Ctrl Pts',(-199.04462738396,-76.0304050557256,8.66757160750338));
#29802=CARTESIAN_POINT('Ctrl Pts',(-198.495170194593,-76.9514494573883,
8.56045714791773));
#29803=CARTESIAN_POINT('Ctrl Pts',(-197.934867869998,-77.8679119426739,
8.4431542477302));
#29804=CARTESIAN_POINT('Ctrl Pts',(-197.366984648206,-78.774595256871,8.31422453249778));
#29805=CARTESIAN_POINT('Ctrl Pts',(-197.339723045589,-78.8181211778033,
8.30803517784311));
#29806=CARTESIAN_POINT('Ctrl Pts',(-197.312442324506,-78.8616273411525,
8.3018195528268));
#29807=CARTESIAN_POINT('Ctrl Pts',(-197.285142554208,-78.9051136828285,
8.29557729592201));
#29808=CARTESIAN_POINT('Ctrl Pts',(-196.511404555994,-80.137616176096,8.11865744241741));
#29809=CARTESIAN_POINT('Ctrl Pts',(-195.722291287618,-81.3543114637074,
7.9204388246629));
#29810=CARTESIAN_POINT('Ctrl Pts',(-194.919125290429,-82.5541339329256,
7.6927527053575));
#29811=CARTESIAN_POINT('Ctrl Pts',(-194.513820130131,-83.1596055787834,
7.57785446588325));
#29812=CARTESIAN_POINT('Ctrl Pts',(-194.104936475455,-83.7607805724009,
7.4554528637455));
#29813=CARTESIAN_POINT('Ctrl Pts',(-193.692644953243,-84.357522691569,7.32450325257206));
#29814=CARTESIAN_POINT('Ctrl Pts',(-193.663328910817,-84.3999541177332,
7.31519206340129));
#29815=CARTESIAN_POINT('Ctrl Pts',(-193.633995705816,-84.4423630558444,
7.30583712450649));
#29816=CARTESIAN_POINT('Ctrl Pts',(-193.604645446565,-84.4847494063933,
7.29643769926986));
#29817=CARTESIAN_POINT('Ctrl Pts',(-193.078197563812,-85.245022231026,7.12784268030665));
#29818=CARTESIAN_POINT('Ctrl Pts',(-192.546256337125,-85.9980368951714,
6.94500033050956));
#29819=CARTESIAN_POINT('Ctrl Pts',(-192.009466142117,-86.7431938561752,
6.74358010351907));
#29820=CARTESIAN_POINT('Ctrl Pts',(-191.933679675978,-86.8483984842011,
6.71514268540938));
#29821=CARTESIAN_POINT('Ctrl Pts',(-191.857796564122,-86.9534464826587,
6.68633503791277));
#29822=CARTESIAN_POINT('Ctrl Pts',(-191.781818629018,-87.0583361629943,
6.65714506117598));
#29823=CARTESIAN_POINT('Ctrl Pts',(-191.751898900846,-87.0996411908201,
6.64565019535609));
#29824=CARTESIAN_POINT('Ctrl Pts',(-191.721964360627,-87.1409217835338,
6.63409686904724));
#29825=CARTESIAN_POINT('Ctrl Pts',(-191.692015202936,-87.18217774886,6.62248370548136));
#29826=CARTESIAN_POINT('Ctrl Pts',(-191.195374169802,-87.8663173648707,
6.42990488203561));
#29827=CARTESIAN_POINT('Ctrl Pts',(-190.694704232015,-88.543696874684,6.22095419572538));
#29828=CARTESIAN_POINT('Ctrl Pts',(-190.190903445975,-89.2134269624852,
5.98937558717201));
#29829=CARTESIAN_POINT('Ctrl Pts',(-190.070696200683,-89.3732250635884,
5.93412075753689));
#29830=CARTESIAN_POINT('Ctrl Pts',(-189.950310726361,-89.532587696832,5.87757794136475));
#29831=CARTESIAN_POINT('Ctrl Pts',(-189.829759241515,-89.6915028144458,
5.81966261655487));
#29832=CARTESIAN_POINT('Ctrl Pts',(-189.799710055655,-89.7311146857652,
5.80522639155477));
#29833=CARTESIAN_POINT('Ctrl Pts',(-189.769650680631,-89.770698618002,5.79070392907296));
#29834=CARTESIAN_POINT('Ctrl Pts',(-189.739581445364,-89.8102542734329,
5.77609284254298));
#29835=CARTESIAN_POINT('Ctrl Pts',(-189.48051683526,-90.151050118778,5.65020951356901));
#29836=CARTESIAN_POINT('Ctrl Pts',(-189.22065314064,-90.4898340171211,5.51773372111318));
#29837=CARTESIAN_POINT('Ctrl Pts',(-188.960371102286,-90.8261693459455,
5.37721625555611));
#29838=CARTESIAN_POINT('Ctrl Pts',(-188.920798880827,-90.8773044000617,
5.35585255216331));
#29839=CARTESIAN_POINT('Ctrl Pts',(-188.881216995801,-90.9283828777641,
5.33430306200019));
#29840=CARTESIAN_POINT('Ctrl Pts',(-188.841626791297,-90.9794032692678,
5.31256280209118));
#29841=CARTESIAN_POINT('Ctrl Pts',(-188.811784559938,-91.0178613259103,
5.29617546905901));
#29842=CARTESIAN_POINT('Ctrl Pts',(-188.781930263047,-91.0562954959819,
5.27967549520592));
#29843=CARTESIAN_POINT('Ctrl Pts',(-188.752067771096,-91.094701048084,5.26306128947281));
#29844=CARTESIAN_POINT('Ctrl Pts',(-188.541474345477,-91.3655410299928,
5.14589616792414));
#29845=CARTESIAN_POINT('Ctrl Pts',(-188.330252784274,-91.6352404391924,
5.02295648219355));
#29846=CARTESIAN_POINT('Ctrl Pts',(-188.119833342626,-91.9020407097296,
4.8936803057521));
#29847=CARTESIAN_POINT('Ctrl Pts',(-188.02973359339,-92.0162822326764,4.83832538707953));
#29848=CARTESIAN_POINT('Ctrl Pts',(-187.939780930582,-92.1299923331076,
4.78180927034326));
#29849=CARTESIAN_POINT('Ctrl Pts',(-187.850087343075,-92.2430339968832,
4.72409069046544));
#29850=CARTESIAN_POINT('Ctrl Pts',(-187.820954449995,-92.2797504533881,
4.70534342811248));
#29851=CARTESIAN_POINT('Ctrl Pts',(-187.791845691714,-92.3164006214176,
4.68646975713368));
#29852=CARTESIAN_POINT('Ctrl Pts',(-187.762763236003,-92.3529821561108,
4.66746483777612));
#29853=CARTESIAN_POINT('Ctrl Pts',(-187.563248765946,-92.6039425832705,
4.53708532472098));
#29854=CARTESIAN_POINT('Ctrl Pts',(-187.364884238019,-92.8517833155242,
4.40057063569385));
#29855=CARTESIAN_POINT('Ctrl Pts',(-187.168269560478,-93.0958704985984,
4.25621167985531));
#29856=CARTESIAN_POINT('Ctrl Pts',(-187.069597876729,-93.2183664060079,
4.18376469158894));
#29857=CARTESIAN_POINT('Ctrl Pts',(-186.971366884062,-93.339917021235,4.10934282074714));
#29858=CARTESIAN_POINT('Ctrl Pts',(-186.873652225136,-93.4604426826047,
4.03273507861638));
#29859=CARTESIAN_POINT('Ctrl Pts',(-186.846241351334,-93.4942524889327,
4.01124510797255));
#29860=CARTESIAN_POINT('Ctrl Pts',(-186.818869584361,-93.5279833711846,
3.98958788461428));
#29861=CARTESIAN_POINT('Ctrl Pts',(-186.79154037738,-93.5616315776803,3.96775330026969));
#29862=CARTESIAN_POINT('Ctrl Pts',(-186.644952825736,-93.7421127826717,
3.85063763487754));
#29863=CARTESIAN_POINT('Ctrl Pts',(-186.499520947913,-93.9202997456518,
3.72843956140678));
#29864=CARTESIAN_POINT('Ctrl Pts',(-186.35585082079,-94.0955230792172,3.59967230248097));
#29865=CARTESIAN_POINT('Ctrl Pts',(-186.222513907549,-94.2581437916332,
3.48016639561181));
#29866=CARTESIAN_POINT('Ctrl Pts',(-186.090694643596,-94.4182116806052,
3.35500174419214));
#29867=CARTESIAN_POINT('Ctrl Pts',(-185.960868132876,-94.5752059646028,
3.22303145109493));
#29868=CARTESIAN_POINT('Ctrl Pts',(-185.950806964742,-94.5873725542976,
3.21280414620755));
#29869=CARTESIAN_POINT('Ctrl Pts',(-185.940757758819,-94.5995206928895,
3.202535992431));
#29870=CARTESIAN_POINT('Ctrl Pts',(-185.930720733152,-94.6116501423323,
3.19222646869787));
#29871=CARTESIAN_POINT('Ctrl Pts',(-185.906249241296,-94.6412232183741,
3.16709059334336));
#29872=CARTESIAN_POINT('Ctrl Pts',(-185.881838142642,-94.6706996607867,
3.1416885525429));
#29873=CARTESIAN_POINT('Ctrl Pts',(-185.857500658255,-94.7000641881417,
3.11601154655574));
#29874=CARTESIAN_POINT('Ctrl Pts',(-185.771154483368,-94.8042456464287,
3.0249129262427));
#29875=CARTESIAN_POINT('Ctrl Pts',(-185.685591537568,-94.9071911396622,
2.9302311934868));
#29876=CARTESIAN_POINT('Ctrl Pts',(-185.601495312243,-95.0081045961674,
2.83162446606724));
#29877=CARTESIAN_POINT('Ctrl Pts',(-185.561162176427,-95.0565033932728,
2.78433199230926));
#29878=CARTESIAN_POINT('Ctrl Pts',(-185.521166286726,-95.1044349798528,
2.73613731470135));
#29879=CARTESIAN_POINT('Ctrl Pts',(-185.481581840516,-95.1518132058979,
2.68700663088748));
#29880=CARTESIAN_POINT('Ctrl Pts',(-185.459407567479,-95.1783533705557,
2.65948478072513));
#29881=CARTESIAN_POINT('Ctrl Pts',(-185.437390340001,-95.2046865189509,
2.63170922282642));
#29882=CARTESIAN_POINT('Ctrl Pts',(-185.415543190754,-95.2307980905917,
2.60366497338433));
#29883=CARTESIAN_POINT('Ctrl Pts',(-185.32184962202,-95.3427800386538,2.48339455352382));
#29884=CARTESIAN_POINT('Ctrl Pts',(-185.231198988516,-95.4507885299479,
2.35812769161362));
#29885=CARTESIAN_POINT('Ctrl Pts',(-185.14448741561,-95.5538311784959,2.22653883183237));
#29886=CARTESIAN_POINT('Ctrl Pts',(-185.118496003256,-95.5847177588987,
2.18709565024665));
#29887=CARTESIAN_POINT('Ctrl Pts',(-185.092858368683,-95.615158333568,2.14708472715111));
#29888=CARTESIAN_POINT('Ctrl Pts',(-185.067598271939,-95.6451266185791,
2.10647110827528));
#29889=CARTESIAN_POINT('Ctrl Pts',(-185.04926100973,-95.6668817332094,2.07698814207058));
#29890=CARTESIAN_POINT('Ctrl Pts',(-185.03112473284,-95.6883856466966,2.04718432923131));
#29891=CARTESIAN_POINT('Ctrl Pts',(-185.013204603834,-95.7096213333921,
2.01703659106574));
#29892=CARTESIAN_POINT('Ctrl Pts',(-184.967811845906,-95.7634125971293,
1.94067056824769));
#29893=CARTESIAN_POINT('Ctrl Pts',(-184.923807018128,-95.8154815879584,
1.86210666755521));
#29894=CARTESIAN_POINT('Ctrl Pts',(-184.881431917216,-95.8655570274556,
1.7809702719163));
#29895=CARTESIAN_POINT('Ctrl Pts',(-184.825774386239,-95.9313285599137,
1.67440175982982));
#29896=CARTESIAN_POINT('Ctrl Pts',(-184.772670985349,-95.9939632911766,
1.56273012066443));
#29897=CARTESIAN_POINT('Ctrl Pts',(-184.724064910961,-96.0512115684829,
1.4475706170276));
#29898=CARTESIAN_POINT('Ctrl Pts',(-184.720923170051,-96.0549119136995,
1.44012707569359));
#29899=CARTESIAN_POINT('Ctrl Pts',(-184.717800207441,-96.0585897677374,
1.43266895612795));
#29900=CARTESIAN_POINT('Ctrl Pts',(-184.714696543205,-96.0622445285302,
1.42519669190371));
#29901=CARTESIAN_POINT('Ctrl Pts',(-184.701735849836,-96.0775065641012,
1.39399301843432));
#29902=CARTESIAN_POINT('Ctrl Pts',(-184.689100103647,-96.0923796827891,
1.36253068298622));
#29903=CARTESIAN_POINT('Ctrl Pts',(-184.676807280731,-96.1068436897848,
1.33079541527949));
#29904=CARTESIAN_POINT('Ctrl Pts',(-184.648777871197,-96.1398237122238,
1.2584344269732));
#29905=CARTESIAN_POINT('Ctrl Pts',(-184.622509882575,-96.1707019647372,
1.18459919006109));
#29906=CARTESIAN_POINT('Ctrl Pts',(-184.598256545621,-96.199191795093,1.10925148363532));
#29907=CARTESIAN_POINT('Ctrl Pts',(-184.591076176966,-96.2076264070098,
1.08694427244499));
#29908=CARTESIAN_POINT('Ctrl Pts',(-184.584072197339,-96.215851904591,1.06450464915634));
#29909=CARTESIAN_POINT('Ctrl Pts',(-184.577250656738,-96.223861464087,1.04193203820146));
#29910=CARTESIAN_POINT('Ctrl Pts',(-184.567880266697,-96.2348637729396,
1.01092523471116));
#29911=CARTESIAN_POINT('Ctrl Pts',(-184.558842564639,-96.2454721860925,
0.979605139691351));
#29912=CARTESIAN_POINT('Ctrl Pts',(-184.550167600447,-96.2556521479711,
0.948014981072279));
#29913=CARTESIAN_POINT('Ctrl Pts',(-184.530838587854,-96.2783345022721,
0.877627765602832));
#29914=CARTESIAN_POINT('Ctrl Pts',(-184.513235022002,-96.2989782309101,
0.805566052494168));
#29915=CARTESIAN_POINT('Ctrl Pts',(-184.497723350323,-96.3171609179611,
0.732331144455422));
#29916=CARTESIAN_POINT('Ctrl Pts',(-184.490400627877,-96.3257445686055,
0.697758538997906));
#29917=CARTESIAN_POINT('Ctrl Pts',(-184.483543702019,-96.3337802274136,
0.662924800421288));
#29918=CARTESIAN_POINT('Ctrl Pts',(-184.477188558001,-96.3412264732102,
0.627883924123101));
#29919=CARTESIAN_POINT('Ctrl Pts',(-184.471708935196,-96.3476468813324,
0.597670480605272));
#29920=CARTESIAN_POINT('Ctrl Pts',(-184.466612404099,-96.3536174294331,
0.567383947479514));
#29921=CARTESIAN_POINT('Ctrl Pts',(-184.461905304076,-96.3591310153293,
0.537033589087389));
#29922=CARTESIAN_POINT('Ctrl Pts',(-184.449891188881,-96.3732035559132,
0.459569184206443));
#29923=CARTESIAN_POINT('Ctrl Pts',(-184.440391292081,-96.3843258397573,
0.381489330036032));
#29924=CARTESIAN_POINT('Ctrl Pts',(-184.433518360913,-96.3923711200197,
0.30289407795958));
#29925=CARTESIAN_POINT('Ctrl Pts',(-184.430352686432,-96.3960767788994,
0.266693077589362));
#29926=CARTESIAN_POINT('Ctrl Pts',(-184.42774387211,-96.3991301793696,0.230382778870197));
#29927=CARTESIAN_POINT('Ctrl Pts',(-184.425700498251,-96.4015217872293,
0.193973205371186));
#29928=CARTESIAN_POINT('Ctrl Pts',(-184.424156021588,-96.4033294752903,
0.166453162295789));
#29929=CARTESIAN_POINT('Ctrl Pts',(-184.422942837909,-96.4047494377422,
0.138819434141523));
#29930=CARTESIAN_POINT('Ctrl Pts',(-184.422059032266,-96.4057838996397,
0.111126891478164));
#29931=CARTESIAN_POINT('Ctrl Pts',(-184.419627274872,-96.4086301819538,
0.0349319203504133));
#29932=CARTESIAN_POINT('Ctrl Pts',(-184.41972428653,-96.4085168258584,-0.0420689086660848));
#29933=CARTESIAN_POINT('Ctrl Pts',(-184.422335964684,-96.4054599928347,
-0.1187107551091));
#29934=CARTESIAN_POINT('Ctrl Pts',(-184.423832696895,-96.4037081458698,
-0.162633594540406));
#29935=CARTESIAN_POINT('Ctrl Pts',(-184.426154715286,-96.4009902805694,
-0.206438375012906));
#29936=CARTESIAN_POINT('Ctrl Pts',(-184.429294421096,-96.3973152254108,
-0.249907542783699));
#29937=CARTESIAN_POINT('Ctrl Pts',(-184.43102093474,-96.3952943249645,-0.27381109164313));
#29938=CARTESIAN_POINT('Ctrl Pts',(-184.432987420065,-96.392992489407,-0.297635627135412));
#29939=CARTESIAN_POINT('Ctrl Pts',(-184.435188366514,-96.3904160126184,
-0.32137898897374));
#29940=CARTESIAN_POINT('Ctrl Pts',(-184.446492157098,-96.3771835443468,
-0.443321978554948));
#29941=CARTESIAN_POINT('Ctrl Pts',(-184.464046436611,-96.3566295002806,
-0.56334586016209));
#29942=CARTESIAN_POINT('Ctrl Pts',(-184.487349843213,-96.3293193460245,
-0.681667501810756));
#29943=CARTESIAN_POINT('Ctrl Pts',(-184.5093818415,-96.3034992038428,-0.793533644414358));
#29944=CARTESIAN_POINT('Ctrl Pts',(-184.53663767668,-96.2715388325085,-0.903702267157027));
#29945=CARTESIAN_POINT('Ctrl Pts',(-184.567717622243,-96.2350535477655,
-1.00994570050335));
#29946=CARTESIAN_POINT('Ctrl Pts',(-184.575817771746,-96.2255446424004,
-1.0376351857431));
#29947=CARTESIAN_POINT('Ctrl Pts',(-184.584177636599,-96.2157284231754,
-1.06505779204202));
#29948=CARTESIAN_POINT('Ctrl Pts',(-184.592772335258,-96.205633599054,-1.09217348702855));
#29949=CARTESIAN_POINT('Ctrl Pts',(-184.59770543273,-96.1998394748694,-1.10773707706353));
#29950=CARTESIAN_POINT('Ctrl Pts',(-184.602718567273,-96.1939504226047,
-1.12322340746622));
#29951=CARTESIAN_POINT('Ctrl Pts',(-184.607810241802,-96.1879681162283,
-1.13863412730332));
#29952=CARTESIAN_POINT('Ctrl Pts',(-184.668299868327,-96.1168976901068,
-1.32171509253029));
#29953=CARTESIAN_POINT('Ctrl Pts',(-184.739770298932,-96.0327883494803,
-1.49401273636365));
#29954=CARTESIAN_POINT('Ctrl Pts',(-184.819572872681,-95.9386084441054,
-1.65829837259598));
#29955=CARTESIAN_POINT('Ctrl Pts',(-184.845731358824,-95.907737212339,-1.71214956231442));
#29956=CARTESIAN_POINT('Ctrl Pts',(-184.872784849862,-95.8757841932931,
-1.76513991495109));
#29957=CARTESIAN_POINT('Ctrl Pts',(-184.90063911685,-95.8428549126627,-1.81736734120617));
#29958=CARTESIAN_POINT('Ctrl Pts',(-184.905815155924,-95.8367358055509,
-1.82707254002346));
#29959=CARTESIAN_POINT('Ctrl Pts',(-184.911017482247,-95.830584581261,-1.83674716358283));
#29960=CARTESIAN_POINT('Ctrl Pts',(-184.916245538324,-95.8244018761813,
-1.846391346213));
#29961=CARTESIAN_POINT('Ctrl Pts',(-185.010656252192,-95.7127516582894,
-2.0205505658697));
#29962=CARTESIAN_POINT('Ctrl Pts',(-185.113242298276,-95.5910902796965,
-2.18442406995139));
#29963=CARTESIAN_POINT('Ctrl Pts',(-185.220589772618,-95.4633228719102,
-2.33893888316464));
#29964=CARTESIAN_POINT('Ctrl Pts',(-185.244425496704,-95.4349530504696,
-2.37324777098454));
#29965=CARTESIAN_POINT('Ctrl Pts',(-185.268495907553,-95.4062822457651,
-2.40709506849083));
#29966=CARTESIAN_POINT('Ctrl Pts',(-185.292763461497,-95.3773533811576,
-2.44049063423734));
#29967=CARTESIAN_POINT('Ctrl Pts',(-185.297183559142,-95.3720842713572,
-2.44657330997149));
#29968=CARTESIAN_POINT('Ctrl Pts',(-185.301611885068,-95.366804592938,-2.45264320377738));
#29969=CARTESIAN_POINT('Ctrl Pts',(-185.306048293262,-95.3615145142168,
-2.45870035369677));
#29970=CARTESIAN_POINT('Ctrl Pts',(-185.39589785598,-95.2543757571472,-2.58137442868812));
#29971=CARTESIAN_POINT('Ctrl Pts',(-185.489079189921,-95.1429511391231,
-2.69884780436733));
#29972=CARTESIAN_POINT('Ctrl Pts',(-185.584265363415,-95.0287750048282,
-2.8113126906656));
#29973=CARTESIAN_POINT('Ctrl Pts',(-185.632328822657,-94.9711227242958,
-2.86810089088767));
#29974=CARTESIAN_POINT('Ctrl Pts',(-185.680902921176,-94.9127695458924,
-2.92361258261388));
#29975=CARTESIAN_POINT('Ctrl Pts',(-185.729814376138,-94.8539160603576,
-2.97787532426895));
#29976=CARTESIAN_POINT('Ctrl Pts',(-185.733340520173,-94.8496731715065,
-2.98178725538923));
#29977=CARTESIAN_POINT('Ctrl Pts',(-185.736868345131,-94.8454277768882,
-2.98569267661173));
#29978=CARTESIAN_POINT('Ctrl Pts',(-185.7403978352,-94.841179894217,-2.98959162660715));
#29979=CARTESIAN_POINT('Ctrl Pts',(-185.887261623273,-94.6644234426887,
-3.15182882080991));
#29980=CARTESIAN_POINT('Ctrl Pts',(-186.037043949676,-94.4833163076637,
-3.30292400819902));
#29981=CARTESIAN_POINT('Ctrl Pts',(-186.1887943239,-94.2989069513012,-3.44588566877327));
#29982=CARTESIAN_POINT('Ctrl Pts',(-186.191461258192,-94.2956660522995,
-3.4483981459717));
#29983=CARTESIAN_POINT('Ctrl Pts',(-186.194128789914,-94.2924241450045,
-3.45090814582523));
#29984=CARTESIAN_POINT('Ctrl Pts',(-186.196796916416,-94.2891812322754,
-3.45341567611537));
#29985=CARTESIAN_POINT('Ctrl Pts',(-186.399577749393,-94.0427159526433,
-3.64399100322999));
#29986=CARTESIAN_POINT('Ctrl Pts',(-186.605788811356,-93.7904494671224,
-3.82032278859053));
#29987=CARTESIAN_POINT('Ctrl Pts',(-186.814296226819,-93.5336032191841,
-3.98595810939003));
#29988=CARTESIAN_POINT('Ctrl Pts',(-186.922152843339,-93.4007419144332,
-4.0716378692109));
#29989=CARTESIAN_POINT('Ctrl Pts',(-187.030623659849,-93.2666554970703,
-4.15445634548737));
#29990=CARTESIAN_POINT('Ctrl Pts',(-187.139550339877,-93.1315149050411,
-4.2349092681681));
#29991=CARTESIAN_POINT('Ctrl Pts',(-187.140897687645,-93.1298433092952,
-4.23590441523151));
#29992=CARTESIAN_POINT('Ctrl Pts',(-187.142245104212,-93.1281715531462,
-4.23689920488079));
#29993=CARTESIAN_POINT('Ctrl Pts',(-187.143592589456,-93.1264996367226,
-4.23789363745222));
#29994=CARTESIAN_POINT('Ctrl Pts',(-187.464496209158,-92.7283327294232,
-4.47471776088121));
#29995=CARTESIAN_POINT('Ctrl Pts',(-187.789269587024,-92.3211070859464,
-4.69128196234316));
#29996=CARTESIAN_POINT('Ctrl Pts',(-188.11636450021,-91.9064086366411,-4.89229634560875));
#29997=CARTESIAN_POINT('Ctrl Pts',(-188.443417007439,-91.491763950584,-5.09328466852566));
#29998=CARTESIAN_POINT('Ctrl Pts',(-188.772790274538,-91.0696485747642,
-5.27872773491933));
#29999=CARTESIAN_POINT('Ctrl Pts',(-189.102923332965,-90.6416650378459,
-5.45338115469171));
#30000=CARTESIAN_POINT('Ctrl Pts',(-189.161372073137,-90.5658411666835,
-5.48418713568767));
#30001=CARTESIAN_POINT('Ctrl Pts',(-188.931799918787,-90.8638551717493,
-6.69061389410879));
#30002=CARTESIAN_POINT('Ctrl Pts',(-189.319051118431,-91.5508432961055,
-7.67806776636097));
#30003=CARTESIAN_POINT('Ctrl Pts',(-188.480882259406,-91.4492167738639,
-5.12686171816464));
#30004=CARTESIAN_POINT('Ctrl Pts',(-188.247114981151,-91.7480740803052,
-6.24241270393816));
#30005=CARTESIAN_POINT('Ctrl Pts',(-188.54325607873,-92.4017170418249,-7.17763983002507));
#30006=CARTESIAN_POINT('Ctrl Pts',(-187.802447662738,-92.3090870122729,
-4.72452254737714));
#30007=CARTESIAN_POINT('Ctrl Pts',(-187.560117152723,-92.6143626232248,
-5.74091658805703));
#30008=CARTESIAN_POINT('Ctrl Pts',(-187.770816940042,-93.2269599088197,
-6.61450397286226));
#30009=CARTESIAN_POINT('Ctrl Pts',(-186.817594622089,-93.5309513688875,
-3.99710358618598));
#30010=CARTESIAN_POINT('Ctrl Pts',(-186.560018651586,-93.8482869695348,
-4.84090069541392));
#30011=CARTESIAN_POINT('Ctrl Pts',(-186.649906375822,-94.3967003926096,
-5.59609535962116));
#30012=CARTESIAN_POINT('Ctrl Pts',(-186.49935620113,-93.9215074314833,-3.73845962749932));
#30013=CARTESIAN_POINT('Ctrl Pts',(-186.237740008661,-94.2416057943953,
-4.52342407349232));
#30014=CARTESIAN_POINT('Ctrl Pts',(-186.287822634423,-94.7700540089429,
-5.2339853240387));
#30015=CARTESIAN_POINT('Ctrl Pts',(-186.033516383533,-94.4876030676821,
-3.29959059467639));
#30016=CARTESIAN_POINT('Ctrl Pts',(-185.765439319798,-94.812289584031,-3.98645759369846));
#30017=CARTESIAN_POINT('Ctrl Pts',(-185.757965731837,-95.3104885264767,
-4.61955372496917));
#30018=CARTESIAN_POINT('Ctrl Pts',(-185.88019021819,-94.6729739327449,-3.14470232538271));
#30019=CARTESIAN_POINT('Ctrl Pts',(-185.610178683132,-94.9989268771276,
-3.79762392135999));
#30020=CARTESIAN_POINT('Ctrl Pts',(-185.58359686481,-95.487331712576,-4.40270469240992));
#30021=CARTESIAN_POINT('Ctrl Pts',(-185.579441491387,-95.0348546295449,
-2.81104162230377));
#30022=CARTESIAN_POINT('Ctrl Pts',(-185.305657248066,-95.3632353428488,
-3.39170158162171));
#30023=CARTESIAN_POINT('Ctrl Pts',(-185.241624386475,-95.8323366660802,
-3.9355677050804));
#30024=CARTESIAN_POINT('Ctrl Pts',(-185.432149758444,-95.2111937660602,
-2.63230461390661));
#30025=CARTESIAN_POINT('Ctrl Pts',(-185.156486831618,-95.5407893224819,
-3.17469909151543));
#30026=CARTESIAN_POINT('Ctrl Pts',(-185.074169959165,-96.0003339135652,
-3.68532933447742));
#30027=CARTESIAN_POINT('Ctrl Pts',(-185.153379734502,-95.5435099326639,
-2.24867201143562));
#30028=CARTESIAN_POINT('Ctrl Pts',(-184.874210151461,-95.8753214389257,
-2.70985007643056));
#30029=CARTESIAN_POINT('Ctrl Pts',(-184.757282758836,-96.3167375829767,
-3.14822934533189));
#30030=CARTESIAN_POINT('Ctrl Pts',(-185.020222521866,-95.7014835433405,
-2.04158414607404));
#30031=CARTESIAN_POINT('Ctrl Pts',(-184.73933109304,-96.0343990644554,-2.45936299143546));
#30032=CARTESIAN_POINT('Ctrl Pts',(-184.60594168315,-96.467044303765,-2.85829845866346));
#30033=CARTESIAN_POINT('Ctrl Pts',(-184.781064427074,-95.9842159788078,
-1.5931390922202));
#30034=CARTESIAN_POINT('Ctrl Pts',(-184.497157491449,-96.3190061700533,
-1.91787402398805));
#30035=CARTESIAN_POINT('Ctrl Pts',(-184.334155197262,-96.7359192863337,
-2.23045805383467));
#30036=CARTESIAN_POINT('Ctrl Pts',(-184.67579092861,-96.1081248174892,-1.3540404464544));
#30037=CARTESIAN_POINT('Ctrl Pts',(-184.390491452695,-96.443809197977,-1.62954253866593));
#30038=CARTESIAN_POINT('Ctrl Pts',(-184.214536143277,-96.853680548758,-1.89571059383307));
#30039=CARTESIAN_POINT('Ctrl Pts',(-184.551305176205,-96.2543384967701,
-0.961207376325233));
#30040=CARTESIAN_POINT('Ctrl Pts',(-184.264389274944,-96.5910392742284,
-1.1563047628428));
#30041=CARTESIAN_POINT('Ctrl Pts',(-184.073096480939,-96.9925975894506,
-1.34572877555771));
#30042=CARTESIAN_POINT('Ctrl Pts',(-184.515191334187,-96.2966908244908,
-0.822876876373191));
#30043=CARTESIAN_POINT('Ctrl Pts',(-184.227811011248,-96.6336802570244,
-0.989790943527011));
#30044=CARTESIAN_POINT('Ctrl Pts',(-184.032066276688,-97.0328274290813,
-1.15206057370444));
#30045=CARTESIAN_POINT('Ctrl Pts',(-184.459543757323,-96.3619063746552,
-0.540441124341592));
#30046=CARTESIAN_POINT('Ctrl Pts',(-184.17146012754,-96.6993255241945,-0.649971919835621));
#30047=CARTESIAN_POINT('Ctrl Pts',(-183.968844518678,-97.094768498995,-0.756639241730944));
#30048=CARTESIAN_POINT('Ctrl Pts',(-184.439877210306,-96.384927969357,-0.3966207303986));
#30049=CARTESIAN_POINT('Ctrl Pts',(-184.151539311701,-96.7225052514127,
-0.476968102648842));
#30050=CARTESIAN_POINT('Ctrl Pts',(-183.94650199697,-97.1166305263899,-0.555284933855703));
#30051=CARTESIAN_POINT('Ctrl Pts',(-184.418726617447,-96.4096849406706,
-0.103191726055235));
#30052=CARTESIAN_POINT('Ctrl Pts',(-184.13012131677,-96.7474252069729,-0.124096554342044));
#30053=CARTESIAN_POINT('Ctrl Pts',(-183.922473553532,-97.1401402657989,
-0.144472556946369));
#30054=CARTESIAN_POINT('Ctrl Pts',(-184.417514594902,-96.4111027446528,
0.0472614384591417));
#30055=CARTESIAN_POINT('Ctrl Pts',(-184.128893590219,-96.7488527806606,
0.0568388822194814));
#30056=CARTESIAN_POINT('Ctrl Pts',(-183.921096645597,-97.1414865203694,
0.0661679095530208));
#30057=CARTESIAN_POINT('Ctrl Pts',(-184.433928343805,-96.3918917393423,
0.340679262061748));
#30058=CARTESIAN_POINT('Ctrl Pts',(-184.145514858577,-96.7295153091363,
0.409686266430749));
#30059=CARTESIAN_POINT('Ctrl Pts',(-183.939743681783,-97.1232435467616,
0.476964636235577));
#30060=CARTESIAN_POINT('Ctrl Pts',(-184.451318549818,-96.3715380527475,
0.485263899435256));
#30061=CARTESIAN_POINT('Ctrl Pts',(-184.163130050764,-96.7090216702262,
0.58359947105962));
#30062=CARTESIAN_POINT('Ctrl Pts',(-183.959500024897,-97.1039154961823,
0.679388918539565));
#30063=CARTESIAN_POINT('Ctrl Pts',(-184.503065282061,-96.3109070247479,
0.770500979869548));
#30064=CARTESIAN_POINT('Ctrl Pts',(-184.215530826723,-96.6479911950592,
0.926759235444962));
#30065=CARTESIAN_POINT('Ctrl Pts',(-184.018289586001,-97.0463305526287,
1.07873223115544));
#30066=CARTESIAN_POINT('Ctrl Pts',(-184.537197371241,-96.2708903134169,
0.909351028970219));
#30067=CARTESIAN_POINT('Ctrl Pts',(-184.250102220423,-96.6077014142732,
1.09388043094421));
#30068=CARTESIAN_POINT('Ctrl Pts',(-184.057067888501,-97.0083208724158,
1.27312782793969));
#30069=CARTESIAN_POINT('Ctrl Pts',(-184.617313485274,-96.1768214097042,
1.17450600394552));
#30070=CARTESIAN_POINT('Ctrl Pts',(-184.331230366073,-96.5130118325845,
1.41315289922425));
#30071=CARTESIAN_POINT('Ctrl Pts',(-184.148094181734,-96.9189506155886,
1.64435530785332));
#30072=CARTESIAN_POINT('Ctrl Pts',(-184.663509817147,-96.1225201391488,
1.30195095812244));
#30073=CARTESIAN_POINT('Ctrl Pts',(-184.378018762994,-96.4583417814738,
1.56670202993));
#30074=CARTESIAN_POINT('Ctrl Pts',(-184.200583375354,-96.8673534301572,
1.82278327080832));
#30075=CARTESIAN_POINT('Ctrl Pts',(-184.765892134559,-96.0019584784386,
1.54843340014367));
#30076=CARTESIAN_POINT('Ctrl Pts',(-184.481693345806,-96.3369830067698,
1.86384266651038));
#30077=CARTESIAN_POINT('Ctrl Pts',(-184.316918986678,-96.7527656506066,
2.16786835852121));
#30078=CARTESIAN_POINT('Ctrl Pts',(-184.822258965331,-95.9354828021284,
1.66765797593972));
#30079=CARTESIAN_POINT('Ctrl Pts',(-184.538778909602,-96.2700583618635,
2.00767566272329));
#30080=CARTESIAN_POINT('Ctrl Pts',(-184.38097095927,-96.689570118882,2.33478741094054));
#30081=CARTESIAN_POINT('Ctrl Pts',(-184.940610822495,-95.7956242175333,
1.89427491600705));
#30082=CARTESIAN_POINT('Ctrl Pts',(-184.658623126078,-96.1292728064777,
2.28126505316723));
#30083=CARTESIAN_POINT('Ctrl Pts',(-184.515467826532,-96.5565741281235,
2.65205989789117));
#30084=CARTESIAN_POINT('Ctrl Pts',(-185.002889262547,-95.7218966402254,
2.00242188310173));
#30085=CARTESIAN_POINT('Ctrl Pts',(-184.721692402306,-96.0550488275035,
2.41193520152812));
#30086=CARTESIAN_POINT('Ctrl Pts',(-184.58624608764,-96.4864461947272,2.80346980635789));
#30087=CARTESIAN_POINT('Ctrl Pts',(-185.197026331985,-95.4915746624195,
2.31455411749728));
#30088=CARTESIAN_POINT('Ctrl Pts',(-184.918382736524,-95.8230687547819,
2.78959213143254));
#30089=CARTESIAN_POINT('Ctrl Pts',(-184.806894376427,-96.2673020072735,
3.24046678270688));
#30090=CARTESIAN_POINT('Ctrl Pts',(-185.336085584367,-95.3259562568104,
2.50639205883812));
#30091=CARTESIAN_POINT('Ctrl Pts',(-185.05923035822,-95.6562990966472,3.02200207733063));
#30092=CARTESIAN_POINT('Ctrl Pts',(-184.964963155496,-96.1096343126113,
3.50904708677375));
#30093=CARTESIAN_POINT('Ctrl Pts',(-185.627101504566,-94.9776421379489,
2.8675740869709));
#30094=CARTESIAN_POINT('Ctrl Pts',(-185.353902675123,-95.3056561818072,
3.46039964178234));
#30095=CARTESIAN_POINT('Ctrl Pts',(-185.295813082335,-95.7778102261891,
4.01471521208864));
#30096=CARTESIAN_POINT('Ctrl Pts',(-185.777854592945,-94.7963843918386,
3.03519751521752));
#30097=CARTESIAN_POINT('Ctrl Pts',(-185.506567110887,-95.1231570680354,
3.66427460436627));
#30098=CARTESIAN_POINT('Ctrl Pts',(-185.467225951133,-95.6050234038876,
4.24939405589426));
#30099=CARTESIAN_POINT('Ctrl Pts',(-186.236474409762,-94.2421557863911,
3.50623173805454));
#30100=CARTESIAN_POINT('Ctrl Pts',(-185.971545136454,-94.5644641073805,
4.2391615355178));
#30101=CARTESIAN_POINT('Ctrl Pts',(-185.988779734173,-95.0763236040051,
4.90885842617087));
#30102=CARTESIAN_POINT('Ctrl Pts',(-186.552577188049,-93.8564712961017,
3.78096556310273));
#30103=CARTESIAN_POINT('Ctrl Pts',(-186.291689470114,-94.1760351311294,
4.57551417638629));
#30104=CARTESIAN_POINT('Ctrl Pts',(-186.348368737014,-94.7079178118668,
5.29349504960836));
#30105=CARTESIAN_POINT('Ctrl Pts',(-187.194773811378,-93.0643566503644,
4.28435082011719));
#30106=CARTESIAN_POINT('Ctrl Pts',(-186.941883309471,-93.3785228823314,
5.19477666592858));
#30107=CARTESIAN_POINT('Ctrl Pts',(-187.079154956339,-93.950182287929,5.99825056968396));
#30108=CARTESIAN_POINT('Ctrl Pts',(-187.521076674221,-92.6576892683202,
4.51235264699091));
#30109=CARTESIAN_POINT('Ctrl Pts',(-187.272289578896,-92.9689762843847,
5.47665603794965));
#30110=CARTESIAN_POINT('Ctrl Pts',(-187.450589338641,-93.5606283707695,
6.31746005549287));
#30111=CARTESIAN_POINT('Ctrl Pts',(-188.179111216884,-91.8283620827728,
4.93577418367053));
#30112=CARTESIAN_POINT('Ctrl Pts',(-187.938458966174,-92.1339334046923,
6.0029378771628));
#30113=CARTESIAN_POINT('Ctrl Pts',(-188.199887644392,-92.7650449264735,
6.91026231965974));
#30114=CARTESIAN_POINT('Ctrl Pts',(-188.511250209779,-91.4051637127826,
5.13113846602503));
#30115=CARTESIAN_POINT('Ctrl Pts',(-188.274704695279,-91.7077535346966,
6.24708719969882));
#30116=CARTESIAN_POINT('Ctrl Pts',(-188.578215964155,-92.3584957265317,
7.18377754322972));
#30117=CARTESIAN_POINT('Ctrl Pts',(-189.172005963988,-90.553639486457,5.49397424413352));
#30118=CARTESIAN_POINT('Ctrl Pts',(-188.943562752701,-90.8502999646729,
6.70318459853149));
#30119=CARTESIAN_POINT('Ctrl Pts',(-189.331108638081,-91.5393071732205,
7.69175665054725));
#30120=CARTESIAN_POINT('Ctrl Pts',(-189.501522189065,-90.1241962177521,
5.66196658596113));
#30121=CARTESIAN_POINT('Ctrl Pts',(-189.277097989269,-90.4178279861717,
6.91560519707551));
#30122=CARTESIAN_POINT('Ctrl Pts',(-189.706696752647,-91.1255979019193,
7.92694977629545));
#30123=CARTESIAN_POINT('Ctrl Pts',(-190.486239445227,-88.8261079680731,
6.13501898383449));
#30124=CARTESIAN_POINT('Ctrl Pts',(-190.276817167461,-89.1066399409558,
7.51936598512612));
#30125=CARTESIAN_POINT('Ctrl Pts',(-190.829455494059,-89.8733451950527,
8.58923262591312));
#30126=CARTESIAN_POINT('Ctrl Pts',(-191.137549166309,-87.9477683977818,
6.40961295141922));
#30127=CARTESIAN_POINT('Ctrl Pts',(-190.935907302917,-88.2219096053228,
7.87329503257363));
#30128=CARTESIAN_POINT('Ctrl Pts',(-191.572553975477,-89.0237350610749,
8.9736687655578));
#30129=CARTESIAN_POINT('Ctrl Pts',(-192.426096187629,-86.1688927511435,
6.90461427891117));
#30130=CARTESIAN_POINT('Ctrl Pts',(-192.239840939106,-86.4303069194794,
8.52054279716209));
#30131=CARTESIAN_POINT('Ctrl Pts',(-193.043608084131,-87.2985121886298,
9.66667669899339));
#30132=CARTESIAN_POINT('Ctrl Pts',(-193.063383291067,-85.2683028918415,
7.12463735631982));
#30133=CARTESIAN_POINT('Ctrl Pts',(-192.884538179013,-85.5231335814101,
8.81258405161933));
#30134=CARTESIAN_POINT('Ctrl Pts',(-193.771620169991,-86.422849070216,9.97471067331157));
#30135=CARTESIAN_POINT('Ctrl Pts',(-194.951173747053,-82.5359543744168,
7.72418030763633));
#30136=CARTESIAN_POINT('Ctrl Pts',(-194.806418839045,-82.7536742244153,
9.62675633492785));
#30137=CARTESIAN_POINT('Ctrl Pts',(-195.929442725192,-83.7595332915572,
10.8140713899068));
#30138=CARTESIAN_POINT('Ctrl Pts',(-196.177482368031,-80.6737566961289,
8.04415647989996));
#30139=CARTESIAN_POINT('Ctrl Pts',(-196.045620897114,-80.8772001990853,
10.0746117618081));
#30140=CARTESIAN_POINT('Ctrl Pts',(-197.332903494677,-81.9356779296839,
11.2620353059768));
#30141=CARTESIAN_POINT('Ctrl Pts',(-197.961738112988,-77.8250108254079,
8.44922123457211));
#30142=CARTESIAN_POINT('Ctrl Pts',(-197.838189296233,-78.0258804597084,
10.662721491043));
#30143=CARTESIAN_POINT('Ctrl Pts',(-199.377119697722,-79.1331363472436,
11.8291181367819));
#30144=CARTESIAN_POINT('Ctrl Pts',(-198.54807446978,-76.8648659123181,8.57151350105634));
#30145=CARTESIAN_POINT('Ctrl Pts',(-198.430673215286,-77.058817715059,10.8457736874515));
#30146=CARTESIAN_POINT('Ctrl Pts',(-200.049262590727,-78.1865264035749,
12.0003238810597));
#30147=CARTESIAN_POINT('Ctrl Pts',(-199.69669086874,-74.9349603932302,8.79383680879332));
#30148=CARTESIAN_POINT('Ctrl Pts',(-199.591479554328,-75.1150846943871,
11.1873231733843));
#30149=CARTESIAN_POINT('Ctrl Pts',(-201.366657824558,-76.2799025943682,
12.3115686050633));
#30150=CARTESIAN_POINT('Ctrl Pts',(-200.259254660993,-73.9648229368186,
8.89394683892728));
#30151=CARTESIAN_POINT('Ctrl Pts',(-200.15966038367,-74.1381129626944,11.3455724974083));
#30152=CARTESIAN_POINT('Ctrl Pts',(-202.012234149144,-75.3195244447861,
12.4517182455822));
#30153=CARTESIAN_POINT('Ctrl Pts',(-201.911900353393,-71.0391139491143,
9.16677201385288));
#30154=CARTESIAN_POINT('Ctrl Pts',(-201.839869083933,-71.1727960227069,
11.7929874150389));
#30155=CARTESIAN_POINT('Ctrl Pts',(-203.909676512503,-72.417697848325,12.8336586580376));
#30156=CARTESIAN_POINT('Ctrl Pts',(-202.966948680821,-69.0682588598496,
9.31223534270219));
#30157=CARTESIAN_POINT('Ctrl Pts',(-202.903401297136,-69.1888071156211,
12.0477177288761));
#30158=CARTESIAN_POINT('Ctrl Pts',(-205.122271910769,-70.4555661236282,
13.0372964661862));
#30159=CARTESIAN_POINT('Ctrl Pts',(-204.984382623087,-65.0867669085141,
9.55122215802441));
#30160=CARTESIAN_POINT('Ctrl Pts',(-204.939612388158,-65.1801116420663,
12.5011483784476));
#30161=CARTESIAN_POINT('Ctrl Pts',(-207.442952278212,-66.4783823872744,
13.3718543161712));
#30162=CARTESIAN_POINT('Ctrl Pts',(-205.946770795552,-63.0761264005556,
9.64459843557726));
#30163=CARTESIAN_POINT('Ctrl Pts',(-205.908524096743,-63.1571838509651,
12.6978518194603));
#30164=CARTESIAN_POINT('Ctrl Pts',(-208.55104128046,-64.4633260703388,13.5025686131142));
#30165=CARTESIAN_POINT('Ctrl Pts',(-208.695489133502,-56.9854174908883,
9.86749344216803));
#30166=CARTESIAN_POINT('Ctrl Pts',(-208.714440707254,-56.9510842463801,
13.2317085155052));
#30167=CARTESIAN_POINT('Ctrl Pts',(-211.718302688857,-58.3414499489575,
13.8145821321649));
#30168=CARTESIAN_POINT('Ctrl Pts',(-210.343625285675,-52.8466938714345,
9.94066884241106));
#30169=CARTESIAN_POINT('Ctrl Pts',(-210.359356788339,-52.7988261518928,
13.4932979556555));
#30170=CARTESIAN_POINT('Ctrl Pts',(-213.6207465057,-54.1580470864287,13.9170012070984));
#30171=CARTESIAN_POINT('Ctrl Pts',(-213.268421736275,-44.4139346324368,
10.0094381670324));
#30172=CARTESIAN_POINT('Ctrl Pts',(-213.300660782719,-44.3236097006244,
13.9242034321311));
#30173=CARTESIAN_POINT('Ctrl Pts',(-217.000471678509,-45.5970270857608,
14.0132264874685));
#30174=CARTESIAN_POINT('Ctrl Pts',(-214.545123000096,-40.1198955494031,
10.0043954519788));
#30175=CARTESIAN_POINT('Ctrl Pts',(-214.567879102413,-40.0304829990944,
14.0859702100237));
#30176=CARTESIAN_POINT('Ctrl Pts',(-218.477811583319,-41.2193854803596,
14.006142250762));
#30177=CARTESIAN_POINT('Ctrl Pts',(-215.901813979384,-34.6533359908493,
9.97920576186224));
#30178=CARTESIAN_POINT('Ctrl Pts',(-215.908024394789,-34.6277287515398,
14.2483264968055));
#30179=CARTESIAN_POINT('Ctrl Pts',(-220.048870888242,-35.6292883846372,
13.9708493230874));
#30180=CARTESIAN_POINT('Ctrl Pts',(-216.161175736962,-33.5548628771818,
9.97318130845029));
#30181=CARTESIAN_POINT('Ctrl Pts',(-216.167513463505,-33.5274498556477,
14.2791323437868));
#30182=CARTESIAN_POINT('Ctrl Pts',(-220.349283740659,-34.5051513167286,
13.9624098056824));
#30183=CARTESIAN_POINT('Ctrl Pts',(-216.653433306906,-31.3585593368,9.95985565386096));
#30184=CARTESIAN_POINT('Ctrl Pts',(-216.660220044528,-31.3274073221036,
14.3367297864681));
#30185=CARTESIAN_POINT('Ctrl Pts',(-220.919563852235,-32.2560153447119,
13.9437437591944));
#30186=CARTESIAN_POINT('Ctrl Pts',(-216.886667558864,-30.2594147169127,
9.95254907226771));
#30187=CARTESIAN_POINT('Ctrl Pts',(-216.893354457392,-30.2271777338965,
14.3635046211515));
#30188=CARTESIAN_POINT('Ctrl Pts',(-221.189823038788,-31.1296731902609,
13.9335096921047));
#30189=CARTESIAN_POINT('Ctrl Pts',(-217.548036348995,-26.959026649267,9.92956539342116));
#30190=CARTESIAN_POINT('Ctrl Pts',(-217.557469895028,-26.9096587272592,
14.4387837536445));
#30191=CARTESIAN_POINT('Ctrl Pts',(-221.956310708416,-27.7455981308832,
13.9013186781023));
#30192=CARTESIAN_POINT('Ctrl Pts',(-217.93785725504,-24.7548304673619,9.91285560896132));
#30193=CARTESIAN_POINT('Ctrl Pts',(-217.945529771334,-24.7081239842741,
14.4813778884191));
#30194=CARTESIAN_POINT('Ctrl Pts',(-222.408272062777,-25.4828152750478,
13.8779166271282));
#30195=CARTESIAN_POINT('Ctrl Pts',(-218.956084319915,-18.1305693881788,
9.86431151402464));
#30196=CARTESIAN_POINT('Ctrl Pts',(-218.968961981201,-18.0402471088626,
14.5919583080073));
#30197=CARTESIAN_POINT('Ctrl Pts',(-223.589086522611,-18.6763260278863,
13.8099328970237));
#30198=CARTESIAN_POINT('Ctrl Pts',(-219.43355866175,-13.6988539781417,9.83453026559723));
#30199=CARTESIAN_POINT('Ctrl Pts',(-219.437341306434,-13.6472841751431,
14.6400615162957));
#30200=CARTESIAN_POINT('Ctrl Pts',(-224.143198140478,-14.1144924088059,
13.7682283895981));
#30201=CARTESIAN_POINT('Ctrl Pts',(-219.989119888241,-4.80453737519254,
9.79912404538294));
#30202=CARTESIAN_POINT('Ctrl Pts',(-219.990808009853,-4.76842009685111,
14.6969168202861));
#30203=CARTESIAN_POINT('Ctrl Pts',(-224.787967419755,-4.95238819466783,
13.7186471999943));
#30204=CARTESIAN_POINT('Ctrl Pts',(-220.067212631373,-0.341936575327023,
9.79351850253299));
#30205=CARTESIAN_POINT('Ctrl Pts',(-220.067252895393,-0.352942294886242,
14.7045953323717));
#30206=CARTESIAN_POINT('Ctrl Pts',(-224.878634407894,-0.352086946103674,
13.7107976404735));
#30207=CARTESIAN_POINT('Ctrl Pts',(-219.879909693335,6.3755153565872,9.80594542214121));
#30208=CARTESIAN_POINT('Ctrl Pts',(-219.880497380835,6.35920093150428,14.6855459823587));
#30209=CARTESIAN_POINT('Ctrl Pts',(-224.661228872703,6.57039409955349,13.7281995569326));
#30210=CARTESIAN_POINT('Ctrl Pts',(-219.766658024021,8.6185966931961,9.81343805283997));
#30211=CARTESIAN_POINT('Ctrl Pts',(-219.768189961766,8.59324909174053,14.674087697868));
#30212=CARTESIAN_POINT('Ctrl Pts',(-224.529776865697,8.88156586473323,13.7386918030301));
#30213=CARTESIAN_POINT('Ctrl Pts',(-219.519208793803,11.989216125175,9.82890166451564));
#30214=CARTESIAN_POINT('Ctrl Pts',(-219.521220785067,11.9640388382862,14.6486293437786));
#30215=CARTESIAN_POINT('Ctrl Pts',(-224.242610932278,12.3530020325013,13.7603463988469));
#30216=CARTESIAN_POINT('Ctrl Pts',(-219.423742238738,13.1138355507161,9.83475451804771));
#30217=CARTESIAN_POINT('Ctrl Pts',(-219.426178170639,13.0864560589663,14.6387997480619));
#30218=CARTESIAN_POINT('Ctrl Pts',(-224.131827752852,13.5110087439763,13.7685425281566));
#30219=CARTESIAN_POINT('Ctrl Pts',(-219.207901176056,15.3538587218567,9.84754794128088));
#30220=CARTESIAN_POINT('Ctrl Pts',(-219.211013282027,15.3236509834499,14.6164107984345));
#30221=CARTESIAN_POINT('Ctrl Pts',(-223.881381580398,15.8168790115975,13.7864581223482));
#30222=CARTESIAN_POINT('Ctrl Pts',(-219.087434557838,16.4706719074987,9.85449428714415));
#30223=CARTESIAN_POINT('Ctrl Pts',(-219.091012905236,16.438758408704,14.6038650095587));
#30224=CARTESIAN_POINT('Ctrl Pts',(-223.741611655969,16.9661945554948,13.7961856778895));
#30225=CARTESIAN_POINT('Ctrl Pts',(-218.422980077555,22.0388998567845,9.89118647406901));
#30226=CARTESIAN_POINT('Ctrl Pts',(-218.433419066376,21.9590251220096,14.5345785986599));
#30227=CARTESIAN_POINT('Ctrl Pts',(-222.97077617523,22.6944728454244,13.8475694404199));
#30228=CARTESIAN_POINT('Ctrl Pts',(-217.693018709706,26.4429011459421,9.92732876816581));
#30229=CARTESIAN_POINT('Ctrl Pts',(-217.714959019159,26.3354267756488,14.4579318865959));
#30230=CARTESIAN_POINT('Ctrl Pts',(-222.124173803383,27.2186160038052,13.8981845777223));
#30231=CARTESIAN_POINT('Ctrl Pts',(-215.845448226668,35.1520276824801,9.98467680865933));
#30232=CARTESIAN_POINT('Ctrl Pts',(-215.866013311531,35.0590051000879,14.2452448518599));
#30233=CARTESIAN_POINT('Ctrl Pts',(-219.983341103331,36.1431189089753,13.97851024857));
#30234=CARTESIAN_POINT('Ctrl Pts',(-214.727821174011,39.4571485295923,10.0059888635688));
#30235=CARTESIAN_POINT('Ctrl Pts',(-214.759629081728,39.3546193987856,14.1128925867739));
#30236=CARTESIAN_POINT('Ctrl Pts',(-218.689081945027,40.54350160402,14.0083695379852));
#30237=CARTESIAN_POINT('Ctrl Pts',(-212.104461778024,47.9683278252243,9.99106655001064));
#30238=CARTESIAN_POINT('Ctrl Pts',(-212.124917932219,47.9013202094227,13.7573388162155));
#30239=CARTESIAN_POINT('Ctrl Pts',(-215.654940347415,49.2109673894579,13.9875274814399));
#30240=CARTESIAN_POINT('Ctrl Pts',(-210.598749993438,52.1743923065104,9.95531537581287));
#30241=CARTESIAN_POINT('Ctrl Pts',(-210.626152534245,52.1133929267026,13.5405466970593));
#30242=CARTESIAN_POINT('Ctrl Pts',(-213.915067425145,53.4780843735008,13.9375020387498));
#30243=CARTESIAN_POINT('Ctrl Pts',(-208.467801042867,57.3684010647384,9.83445365866558));
#30244=CARTESIAN_POINT('Ctrl Pts',(-208.440496676423,57.4335485585645,13.1675008632595));
#30245=CARTESIAN_POINT('Ctrl Pts',(-211.45675431658,58.7206047789808,13.7683295199504));
#30246=CARTESIAN_POINT('Ctrl Pts',(-208.029146170907,58.4040178152079,9.80639282881666));
#30247=CARTESIAN_POINT('Ctrl Pts',(-207.998880661217,58.4750011351285,13.0896849260068));
#30248=CARTESIAN_POINT('Ctrl Pts',(-210.950890758971,59.7645343781391,13.7290510241888));
#30249=CARTESIAN_POINT('Ctrl Pts',(-207.12664788482,60.4688131192695,9.74108338571404));
#30250=CARTESIAN_POINT('Ctrl Pts',(-207.089446964967,60.5522052555366,12.9231741124707));
#30251=CARTESIAN_POINT('Ctrl Pts',(-209.910535831253,61.8429955994894,13.6376310670489));
#30252=CARTESIAN_POINT('Ctrl Pts',(-206.662970155658,61.4975272274392,9.70383665509011));
#30253=CARTESIAN_POINT('Ctrl Pts',(-206.62229251033,61.587147971588,12.8346671765189));
#30254=CARTESIAN_POINT('Ctrl Pts',(-209.376236001022,62.8770556591804,13.5854922099582));
#30255=CARTESIAN_POINT('Ctrl Pts',(-205.240266007795,64.5604067343896,9.5765196532658));
#30256=CARTESIAN_POINT('Ctrl Pts',(-205.196584633148,64.650427049727,12.5533538086537));
#30257=CARTESIAN_POINT('Ctrl Pts',(-207.737539989063,65.9512466063413,13.4072675873146));
#30258=CARTESIAN_POINT('Ctrl Pts',(-204.247673314577,66.5757395952135,9.47090861845935));
#30259=CARTESIAN_POINT('Ctrl Pts',(-204.196792574619,66.6787164938637,12.3422625706762));
#30260=CARTESIAN_POINT('Ctrl Pts',(-206.595163150902,67.9678447656868,13.259424414464));
#30261=CARTESIAN_POINT('Ctrl Pts',(-202.175877209204,70.5527743625175,9.20351075943804));
#30262=CARTESIAN_POINT('Ctrl Pts',(-202.105162467068,70.6833454593898,11.8563179607818));
#30263=CARTESIAN_POINT('Ctrl Pts',(-204.213034709984,71.9338913959523,12.8850903188223));
#30264=CARTESIAN_POINT('Ctrl Pts',(-201.096663082113,72.5144855502291,9.04188771001516));
#30265=CARTESIAN_POINT('Ctrl Pts',(-201.016769126083,72.6586875911064,11.5835583962009));
#30266=CARTESIAN_POINT('Ctrl Pts',(-202.973270051406,73.8833489271374,12.6588283062611));
#30267=CARTESIAN_POINT('Ctrl Pts',(-198.853190944606,76.3831310032251,8.64078280219066));
#30268=CARTESIAN_POINT('Ctrl Pts',(-198.749688199617,76.5553396176626,10.9496183488417));
#30269=CARTESIAN_POINT('Ctrl Pts',(-200.398794120576,77.7129932538224,12.097299012796));
#30270=CARTESIAN_POINT('Ctrl Pts',(-197.688906293114,78.2900912932045,8.4017397701364));
#30271=CARTESIAN_POINT('Ctrl Pts',(-197.574275171399,78.4761661484505,10.5915528796197));
#30272=CARTESIAN_POINT('Ctrl Pts',(-199.064051750511,79.593204560045,11.7626455547735));
#30273=CARTESIAN_POINT('Ctrl Pts',(-195.880204369929,81.1077158340626,7.95715194188713));
#30274=CARTESIAN_POINT('Ctrl Pts',(-195.7336336546,81.3323663938434,9.95197272056883));
#30275=CARTESIAN_POINT('Ctrl Pts',(-196.992976264055,82.3591154501006,11.1402297609643));
#30276=CARTESIAN_POINT('Ctrl Pts',(-195.266929615523,82.0397774649153,7.79447520511931));
#30277=CARTESIAN_POINT('Ctrl Pts',(-195.113586791239,82.271187103462,9.7241882232041));
#30278=CARTESIAN_POINT('Ctrl Pts',(-196.291129043696,83.2720093140021,10.9124837103213));
#30279=CARTESIAN_POINT('Ctrl Pts',(-194.020039407559,83.8890943957255,7.43221244761711));
#30280=CARTESIAN_POINT('Ctrl Pts',(-193.852340906558,84.1338848996827,9.22650488428313));
#30281=CARTESIAN_POINT('Ctrl Pts',(-194.865016774257,85.0790184789678,10.4053168524648));
#30282=CARTESIAN_POINT('Ctrl Pts',(-193.386270744956,84.8064721381628,7.2325858360569));
#30283=CARTESIAN_POINT('Ctrl Pts',(-193.211305013333,85.0579843658949,8.9571159136994));
#30284=CARTESIAN_POINT('Ctrl Pts',(-194.140578625951,85.9732430528797,10.1258390890344));
#30285=CARTESIAN_POINT('Ctrl Pts',(-192.107819334031,86.61357210353,6.78753527125637));
#30286=CARTESIAN_POINT('Ctrl Pts',(-191.917758060802,86.8780799988377,8.36623872478481));
#30287=CARTESIAN_POINT('Ctrl Pts',(-192.680140055584,87.7303403765514,9.50276493243055));
#30288=CARTESIAN_POINT('Ctrl Pts',(-191.462180488014,87.5047202513877,6.54205946399846));
#30289=CARTESIAN_POINT('Ctrl Pts',(-191.264472823669,87.7757783231601,8.04532402545658));
#30290=CARTESIAN_POINT('Ctrl Pts',(-191.943046059177,88.5946069753687,9.15909579322666));
#30291=CARTESIAN_POINT('Ctrl Pts',(-190.150638039327,89.2738373630881,5.98189948503679));
#30292=CARTESIAN_POINT('Ctrl Pts',(-189.937244247952,89.5572864784185,7.32319343760467));
#30293=CARTESIAN_POINT('Ctrl Pts',(-190.446683438805,90.3058737452788,8.37486245635653));
#30294=CARTESIAN_POINT('Ctrl Pts',(-189.484435938415,90.1514762972045,5.66676146619764));
#30295=CARTESIAN_POINT('Ctrl Pts',(-189.262882995061,90.4414214467756,6.92234530392305));
#30296=CARTESIAN_POINT('Ctrl Pts',(-189.687009990413,91.1525614199763,7.93360765281502));
#30297=CARTESIAN_POINT('Ctrl Pts',(-188.817225428583,91.010840855218,5.29913391686224));
#30298=CARTESIAN_POINT('Ctrl Pts',(-188.583433673891,91.3119644595324,6.4575852679122));
#30299=CARTESIAN_POINT('Ctrl Pts',(-188.926861534792,91.9791409821367,7.41897832366544));
#39945=UNCERTAINTY_MEASURE_WITH_UNIT(LENGTH_MEASURE(0.01),#39960,
'DISTANCE_ACCURACY_VALUE',
'Maximum model space distance between geometric entities at asserted c
onnectivities');
#39950=UNCERTAINTY_MEASURE_WITH_UNIT(LENGTH_MEASURE(0.01),#39960,
'DISTANCE_ACCURACY_VALUE',
'Maximum model space distance between geometric entities at asserted c
onnectivities');
#39954=(
GEOMETRIC_REPRESENTATION_CONTEXT(3)
GLOBAL_UNCERTAINTY_ASSIGNED_CONTEXT((#39945))
GLOBAL_UNIT_ASSIGNED_CONTEXT((#39960,#39962,#39963))
REPRESENTATION_CONTEXT('','3D')
);
#39959=(
GEOMETRIC_REPRESENTATION_CONTEXT(3)
GLOBAL_UNCERTAINTY_ASSIGNED_CONTEXT((#39950))
GLOBAL_UNIT_ASSIGNED_CONTEXT((#39960,#39962,#39963))
REPRESENTATION_CONTEXT('','3D')
);
#39960=(
LENGTH_UNIT()
NAMED_UNIT(*)
SI_UNIT(.MILLI.,.METRE.)
);
#39962=(
NAMED_UNIT(*)
PLANE_ANGLE_UNIT()
SI_UNIT($,.RADIAN.)
);
#39963=(
NAMED_UNIT(*)
SI_UNIT($,.STERADIAN.)
SOLID_ANGLE_UNIT()
);
#39967=SHAPE_DEFINITION_REPRESENTATION(#39975,#40004);
#39975=PRODUCT_DEFINITION_SHAPE('',$,#40013);
#40004=SHAPE_REPRESENTATION('',(#18721),#39954);
#40009=PRODUCT_DEFINITION_CONTEXT('part definition',#40035,'design');
#40013=PRODUCT_DEFINITION('Flexible Tubing','Flexible Tubing',#40021,#40009);
#40021=PRODUCT_DEFINITION_FORMATION('',$,#40040);
#40035=APPLICATION_CONTEXT(
'Core Data for Automotive Mechanical Design Process');
#40036=PRODUCT_CONTEXT('part definition',#40035,'mechanical');
#40040=PRODUCT('Flexible Tubing','Flexible Tubing',$,(#40036));
#40046=PRESENTATION_STYLE_ASSIGNMENT((#40048));
#40048=SURFACE_STYLE_USAGE(.BOTH.,#40050);
#40050=SURFACE_SIDE_STYLE('',(#40052));
#40052=SURFACE_STYLE_FILL_AREA(#40054);
#40054=FILL_AREA_STYLE('Opaque(202,209,238)',(#40056));
#40056=FILL_AREA_STYLE_COLOUR('Opaque(202,209,238)',#40058);
#40058=COLOUR_RGB('Opaque(202,209,238)', 0.66274510, 0.83137255, 0.94901961);
ENDSEC;
END-ISO-10303-21;
